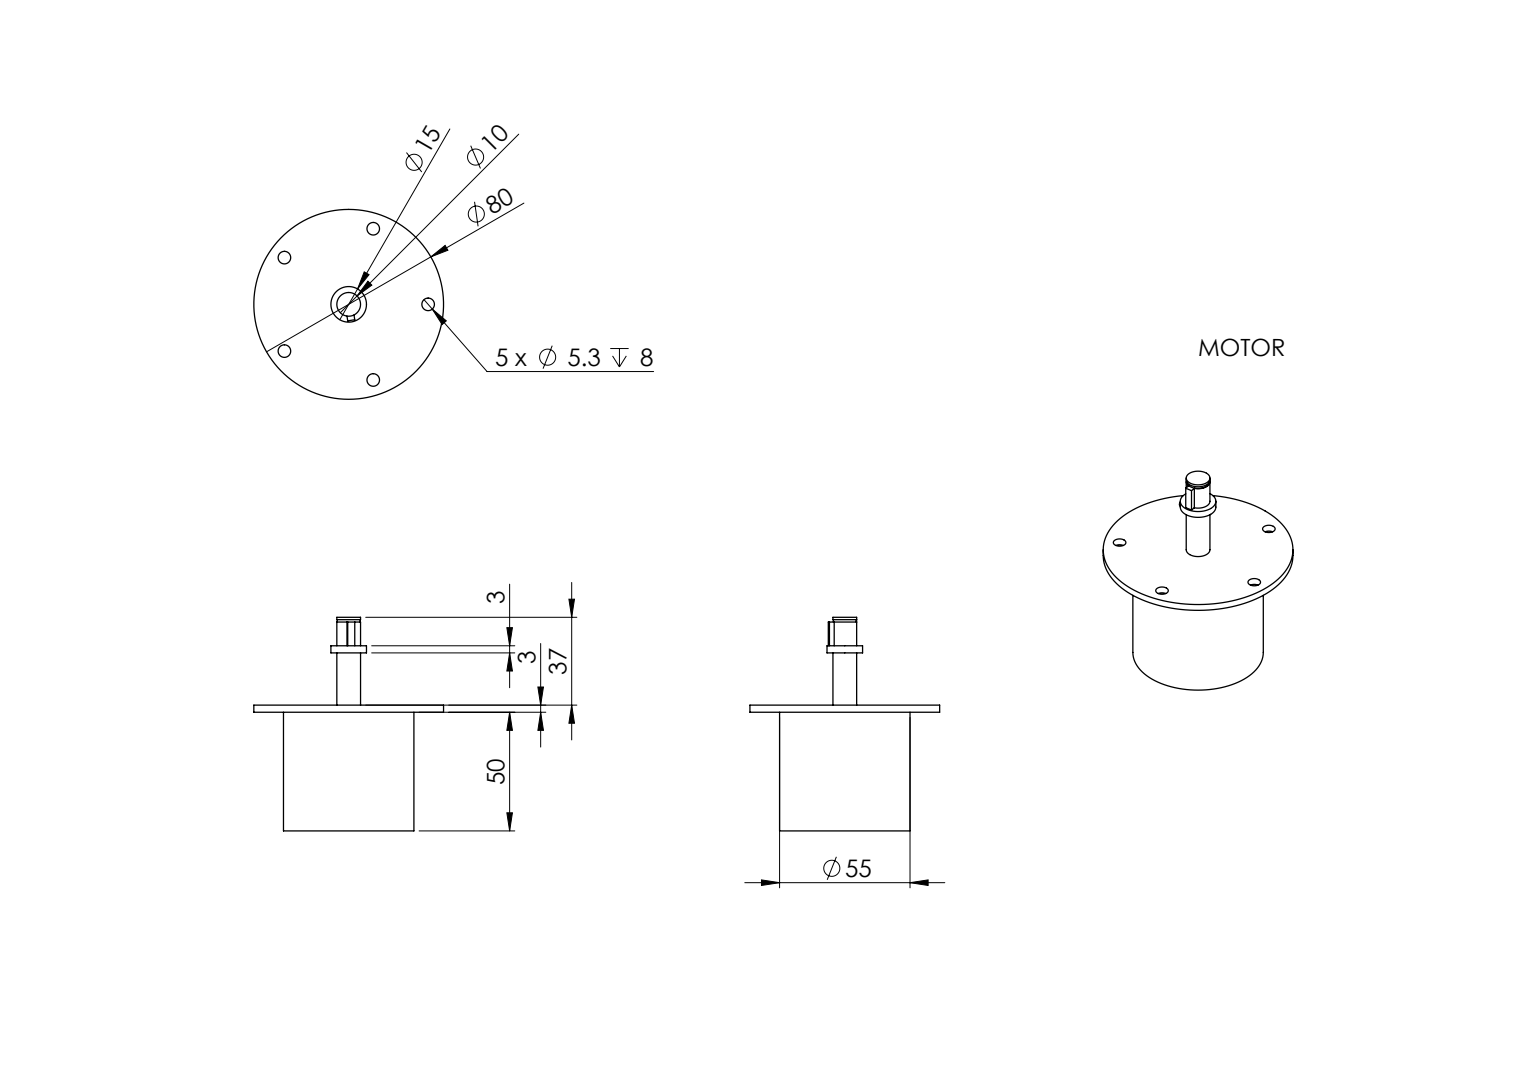
ISO-10303-21;
HEADER;
FILE_DESCRIPTION (('STEP AP214'),
    '1' );
FILE_NAME ('motor.step',
    '2026-10-24T07:08:27',
    ( '' ),
    ( '' ),
    'SwSTEP 2.0',
    'SolidWorks 2026',
    '' );
FILE_SCHEMA (( 'AUTOMOTIVE_DESIGN' ));
ENDSEC;

DATA;
#42=EDGE_CURVE ( 'NONE', #9389, #8733, #2574, .T. ) ;
#55=AXIS2_PLACEMENT_3D ( 'NONE', #9559, #12524, #9279 ) ;
#62=PLANE ( 'NONE',  #8396 ) ;
#84=CARTESIAN_POINT ( 'NONE',  ( -90.00000000009001155, -38.00000000000000000, -1.301042606982603940E-15 ) ) ;
#93=ORIENTED_EDGE ( 'NONE', *, *, #7771, .T. ) ;
#98=FACE_OUTER_BOUND ( 'NONE', #15027, .T. ) ;
#208=DIRECTION ( 'NONE',  ( 0.000000000000000000, 0.000000000000000000, -1.000000000000000000 ) ) ;
#226=CIRCLE ( 'NONE', #3261, 2.649999999999992806 ) ;
#240=CARTESIAN_POINT ( 'NONE',  ( -90.00000000009001155, -38.00000000000000000, -1.301042606982603940E-15 ) ) ;
#245=VECTOR ( 'NONE', #14490, 1000.000000000000000 ) ;
#258=LINE ( 'NONE', #11691, #3125 ) ;
#277=CARTESIAN_POINT ( 'NONE',  ( -90.67999921423555065, 1.000000000000018208, -4.751589320297106234 ) ) ;
#297=AXIS2_PLACEMENT_3D ( 'NONE', #16898, #13842, #16521 ) ;
#342=EDGE_CURVE ( 'NONE', #3837, #6567, #9219, .T. ) ;
#375=EDGE_CURVE ( 'NONE', #12355, #6629, #15146, .T. ) ;
#395=EDGE_CURVE ( 'NONE', #2599, #6420, #1243, .T. ) ;
#405=EDGE_CURVE ( 'NONE', #10887, #2703, #6947, .T. ) ;
#426=ORIENTED_EDGE ( 'NONE', *, *, #405, .T. ) ;
#436=DIRECTION ( 'NONE',  ( 0.000000000000000000, 0.000000000000000000, 1.000000000000000000 ) ) ;
#459=DIRECTION ( 'NONE',  ( 0.000000000000000000, -1.000000000000000000, 0.000000000000000000 ) ) ;
#485=CARTESIAN_POINT ( 'NONE',  ( -90.40159941089927997, 2.081668171172168513E-14, -4.983845695167307355 ) ) ;
#496=EDGE_CURVE ( 'NONE', #11686, #6003, #9891, .T. ) ;
#506=CIRCLE ( 'NONE', #15414, 5.000000000000004441 ) ;
#535=ORIENTED_EDGE ( 'NONE', *, *, #4870, .T. ) ;
#542=VECTOR ( 'NONE', #17182, 1000.000000000000000 ) ;
#547=ORIENTED_EDGE ( 'NONE', *, *, #996, .F. ) ;
#549=LINE ( 'NONE', #1872, #13865 ) ;
#550=ORIENTED_EDGE ( 'NONE', *, *, #5972, .T. ) ;
#563=CARTESIAN_POINT ( 'NONE',  ( -90.00000000009001155, -10.00000000000001599, -1.301042606982603940E-15 ) ) ;
#564=CYLINDRICAL_SURFACE ( 'NONE', #2820, 7.500000000000007105 ) ;
#565=VECTOR ( 'NONE', #11959, 1000.000000000000000 ) ;
#580=EDGE_LOOP ( 'NONE', ( #11778, #1324 ) ) ;
#594=ORIENTED_EDGE ( 'NONE', *, *, #13827, .T. ) ;
#597=CARTESIAN_POINT ( 'NONE',  ( -90.38553543446691663, 1.000000000000018208, -4.784491867360616268 ) ) ;
#598=CARTESIAN_POINT ( 'NONE',  ( -79.64793068852927149, -38.00000000000000000, 34.51039329588763849 ) ) ;
#601=CARTESIAN_POINT ( 'NONE',  ( -90.00000000009001155, -13.00000000000001776, -1.691355389077386325E-15 ) ) ;
#653=ORIENTED_EDGE ( 'NONE', *, *, #10856, .F. ) ;
#671=ORIENTED_EDGE ( 'NONE', *, *, #1460, .F. ) ;
#696=LINE ( 'NONE', #18305, #3229 ) ;
#706=CIRCLE ( 'NONE', #11348, 2.649999999999992806 ) ;
#727=DIRECTION ( 'NONE',  ( 0.000000000000000000, 0.000000000000000000, 1.000000000000000000 ) ) ;
#738=ORIENTED_EDGE ( 'NONE', *, *, #1656, .F. ) ;
#745=STYLED_ITEM ( 'NONE', ( #16686 ), #12609 ) ;
#760=CARTESIAN_POINT ( 'NONE',  ( -94.77031323234206184, 1.000000000000018208, 0.5330212624288541701 ) ) ;
#764=EDGE_CURVE ( 'NONE', #3720, #10887, #3348, .T. ) ;
#776=CARTESIAN_POINT ( 'NONE',  ( -90.00000000009001155, -49.14213562373095812, -5.000000000000005329 ) ) ;
#797=CARTESIAN_POINT ( 'NONE',  ( -90.00000000009001155, -38.00000000000000000, 40.00000000000000000 ) ) ;
#826=UNCERTAINTY_MEASURE_WITH_UNIT (LENGTH_MEASURE( 1.000000000000000082E-05 ), #11317, 'distance_accuracy_value', 'NONE');
#832=CIRCLE ( 'NONE', #6896, 5.000000000000004441 ) ;
#841=AXIS2_PLACEMENT_3D ( 'NONE', #6851, #12669, #4200 ) ;
#846=AXIS2_PLACEMENT_3D ( 'NONE', #6460, #16655, #9411 ) ;
#859=ORIENTED_EDGE ( 'NONE', *, *, #4333, .F. ) ;
#870=AXIS2_PLACEMENT_3D ( 'NONE', #15554, #18308, #10969 ) ;
#874=ORIENTED_EDGE ( 'NONE', *, *, #16459, .T. ) ;
#879=AXIS2_PLACEMENT_3D ( 'NONE', #17078, #7057, #1436 ) ;
#886=CARTESIAN_POINT ( 'NONE',  ( -90.70833251482494575, 2.081668171172168513E-14, -4.949572208642815774 ) ) ;
#892=CIRCLE ( 'NONE', #4521, 2.649999999999992806 ) ;
#913=ORIENTED_EDGE ( 'NONE', *, *, #375, .F. ) ;
#948=ORIENTED_EDGE ( 'NONE', *, *, #9136, .F. ) ;
#949=CARTESIAN_POINT ( 'NONE',  ( -90.00000000009001155, -10.00000000000001599, -1.301042606982603940E-15 ) ) ;
#956=CYLINDRICAL_SURFACE ( 'NONE', #8481, 2.649999999999992806 ) ;
#990=LINE ( 'NONE', #1078, #10722 ) ;
#994=ORIENTED_EDGE ( 'NONE', *, *, #375, .T. ) ;
#996=EDGE_CURVE ( 'NONE', #8916, #9803, #18000, .T. ) ;
#1006=CARTESIAN_POINT ( 'NONE',  ( -117.1020693116506379, -30.00000000000000000, -19.69080595179801207 ) ) ;
#1015=DIRECTION ( 'NONE',  ( 0.000000000000000000, -1.000000000000000000, 0.000000000000000000 ) ) ;
#1020=CARTESIAN_POINT ( 'NONE',  ( -56.50000000009000445, -34.99999999999999289, -2.649999999999610889 ) ) ;
#1075=DIRECTION ( 'NONE',  ( -2.031314180040284764E-16, -1.000000000000000000, -1.301042606982601377E-16 ) ) ;
#1078=CARTESIAN_POINT ( 'NONE',  ( -90.00000000009001155, -49.14213562373095812, -5.000000000000005329 ) ) ;
#1079=DIRECTION ( 'NONE',  ( -0.000000000000000000, 1.000000000000000000, -0.000000000000000000 ) ) ;
#1095=ADVANCED_FACE ( 'NONE', ( #18192 ), #16772, .F. ) ;
#1110=DIRECTION ( 'NONE',  ( 1.000000000000000000, -3.469446951953611231E-16, 0.000000000000000000 ) ) ;
#1121=AXIS2_PLACEMENT_3D ( 'NONE', #7531, #10470, #14766 ) ;
#1127=DIRECTION ( 'NONE',  ( -0.000000000000000000, 1.000000000000000000, 0.000000000000000000 ) ) ;
#1137=DIRECTION ( 'NONE',  ( -1.000000000000000000, 2.312964634635740492E-16, 0.000000000000000000 ) ) ;
#1165=CIRCLE ( 'NONE', #4494, 2.649999999999992806 ) ;
#1174=ORIENTED_EDGE ( 'NONE', *, *, #18088, .F. ) ;
#1182=LINE ( 'NONE', #4037, #9056 ) ;
#1203=CYLINDRICAL_SURFACE ( 'NONE', #14853, 2.649999999999992806 ) ;
#1204=ORIENTED_EDGE ( 'NONE', *, *, #3441, .T. ) ;
#1211=ORIENTED_EDGE ( 'NONE', *, *, #18679, .T. ) ;
#1217=ADVANCED_FACE ( 'NONE', ( #14378 ), #15990, .F. ) ;
#1219=EDGE_CURVE ( 'NONE', #9771, #12239, #15903, .T. ) ;
#1220=CARTESIAN_POINT ( 'NONE',  ( -90.00000000009003998, 1.000000000000018208, -5.746271514173173500E-15 ) ) ;
#1222=CARTESIAN_POINT ( 'NONE',  ( -90.38553543446691663, 1.000000000000018208, -4.784491867360616268 ) ) ;
#1243=LINE ( 'NONE', #7037, #13136 ) ;
#1277=VERTEX_POINT ( 'NONE', #12642 ) ;
#1287=ORIENTED_EDGE ( 'NONE', *, *, #12978, .F. ) ;
#1324=ORIENTED_EDGE ( 'NONE', *, *, #10853, .T. ) ;
#1339=CARTESIAN_POINT ( 'NONE',  ( -90.00000000009003998, 1.000000000000018208, -5.746271514173173500E-15 ) ) ;
#1364=ORIENTED_EDGE ( 'NONE', *, *, #3902, .T. ) ;
#1370=ORIENTED_EDGE ( 'NONE', *, *, #1440, .F. ) ;
#1374=DIRECTION ( 'NONE',  ( 0.000000000000000000, 0.000000000000000000, 1.000000000000000000 ) ) ;
#1382=DIRECTION ( 'NONE',  ( -0.000000000000000000, 1.000000000000000000, -0.000000000000000000 ) ) ;
#1387=DIRECTION ( 'NONE',  ( -2.031314180040284764E-16, -1.000000000000000000, -1.301042606982601377E-16 ) ) ;
#1398=FACE_OUTER_BOUND ( 'NONE', #2904, .T. ) ;
#1402=CYLINDRICAL_SURFACE ( 'NONE', #7880, 7.500000000000007105 ) ;
#1423=CYLINDRICAL_SURFACE ( 'NONE', #16347, 40.00000000000000000 ) ;
#1428=CARTESIAN_POINT ( 'NONE',  ( -90.00000000009001155, -88.00000000000000000, 27.50000000000000000 ) ) ;
#1436=DIRECTION ( 'NONE',  ( 1.000000000000000000, -2.031314180040284764E-16, 0.000000000000000000 ) ) ;
#1440=EDGE_CURVE ( 'NONE', #1277, #9572, #17130, .T. ) ;
#1453=DIRECTION ( 'NONE',  ( -0.000000000000000000, 1.000000000000000000, -0.000000000000000000 ) ) ;
#1456=ORIENTED_EDGE ( 'NONE', *, *, #14822, .T. ) ;
#1460=EDGE_CURVE ( 'NONE', #9528, #7635, #226, .T. ) ;
#1507=VERTEX_POINT ( 'NONE', #9356 ) ;
#1527=CARTESIAN_POINT ( 'NONE',  ( -90.00000000009001155, 2.000000000000001776, -1.301042606982603940E-15 ) ) ;
#1558=FACE_OUTER_BOUND ( 'NONE', #2676, .T. ) ;
#1575=FACE_BOUND ( 'NONE', #4154, .T. ) ;
#1590=CARTESIAN_POINT ( 'NONE',  ( -90.00000000009001155, 2.000000000000001776, -5.000000000000005329 ) ) ;
#1591=DIRECTION ( 'NONE',  ( -0.000000000000000000, 1.000000000000000000, -0.000000000000000000 ) ) ;
#1624=LINE ( 'NONE', #17534, #2968 ) ;
#1645=CARTESIAN_POINT ( 'NONE',  ( -87.43997332177200121, -10.00000000000001954, 6.475821446449875118 ) ) ;
#1656=EDGE_CURVE ( 'NONE', #2709, #2599, #1182, .T. ) ;
#1666=DIRECTION ( 'NONE',  ( 0.1416665029469836024, 0.000000000000000000, 0.9899144417285627995 ) ) ;
#1677=DIRECTION ( 'NONE',  ( -2.031314180040284764E-16, -1.000000000000000000, -1.301042606982601377E-16 ) ) ;
#1681=EDGE_CURVE ( 'NONE', #3221, #14211, #7538, .T. ) ;
#1703=VECTOR ( 'NONE', #11338, 1000.000000000000000 ) ;
#1724=DIRECTION ( 'NONE',  ( 0.000000000000000000, 0.000000000000000000, 1.000000000000000000 ) ) ;
#1737=EDGE_LOOP ( 'NONE', ( #6979, #13598, #3643, #15086 ) ) ;
#1738=FACE_OUTER_BOUND ( 'NONE', #1758, .T. ) ;
#1747=DIRECTION ( 'NONE',  ( 0.1586811557617576196, -1.606889522083438452E-16, 0.9873298794253686506 ) ) ;
#1753=ORIENTED_EDGE ( 'NONE', *, *, #3346, .T. ) ;
#1758=EDGE_LOOP ( 'NONE', ( #16142, #8598, #12894, #6927 ) ) ;
#1761=PRODUCT_DEFINITION_SHAPE ( 'NONE', 'NONE',  #8863 ) ;
#1764=CIRCLE ( 'NONE', #16379, 5.000000000000004441 ) ;
#1770=SHAPE_REPRESENTATION ( 'motor', ( #8017 ), #16855 ) ;
#1775=LINE ( 'NONE', #6150, #565 ) ;
#1791=EDGE_LOOP ( 'NONE', ( #6997, #7591, #14174, #14685 ) ) ;
#1792=EDGE_CURVE ( 'NONE', #10035, #1893, #8740, .T. ) ;
#1793=EDGE_CURVE ( 'NONE', #12173, #10035, #8405, .T. ) ;
#1796=LINE ( 'NONE', #277, #17542 ) ;
#1811=DIRECTION ( 'NONE',  ( 0.000000000000000000, -1.000000000000000000, 0.000000000000000000 ) ) ;
#1816=CYLINDRICAL_SURFACE ( 'NONE', #2469, 2.649999999999992806 ) ;
#1841=DIRECTION ( 'NONE',  ( 0.1416665029469836024, 0.000000000000000000, 0.9899144417285627995 ) ) ;
#1845=EDGE_CURVE ( 'NONE', #1507, #12191, #2986, .T. ) ;
#1867=AXIS2_PLACEMENT_3D ( 'NONE', #14318, #14592, #8682 ) ;
#1872=CARTESIAN_POINT ( 'NONE',  ( -87.43997332177200121, -14.11572627500821042, 6.475821446449874230 ) ) ;
#1875=EDGE_CURVE ( 'NONE', #3186, #11692, #14402, .T. ) ;
#1878=FACE_OUTER_BOUND ( 'NONE', #15547, .T. ) ;
#1893=VERTEX_POINT ( 'NONE', #3072 ) ;
#1906=VECTOR ( 'NONE', #18383, 1000.000000000000000 ) ;
#1909=EDGE_CURVE ( 'NONE', #6825, #12049, #7067, .T. ) ;
#1939=DIRECTION ( 'NONE',  ( 0.000000000000000000, -1.000000000000000000, 0.000000000000000000 ) ) ;
#1958=DIRECTION ( 'NONE',  ( 0.000000000000000000, 0.000000000000000000, 1.000000000000000000 ) ) ;
#1983=PLANE ( 'NONE',  #16615 ) ;
#1991=AXIS2_PLACEMENT_3D ( 'NONE', #7672, #14832, #13501 ) ;
#2033=AXIS2_PLACEMENT_3D ( 'NONE', #1220, #12453, #13874 ) ;
#2039=DIRECTION ( 'NONE',  ( -0.000000000000000000, 1.000000000000000000, -0.000000000000000000 ) ) ;
#2067=ORIENTED_EDGE ( 'NONE', *, *, #7457, .F. ) ;
#2068=AXIS2_PLACEMENT_3D ( 'NONE', #17088, #15644, #2591 ) ;
#2070=DIRECTION ( 'NONE',  ( 0.000000000000000000, 0.000000000000000000, 1.000000000000000000 ) ) ;
#2103=DIRECTION ( 'NONE',  ( -0.000000000000000000, 1.000000000000000000, -0.000000000000000000 ) ) ;
#2124=CARTESIAN_POINT ( 'NONE',  ( -90.67999921423555065, 1.000000000000018208, -4.751589320297106234 ) ) ;
#2132=ORIENTED_EDGE ( 'NONE', *, *, #11827, .T. ) ;
#2149=ORIENTED_EDGE ( 'NONE', *, *, #4870, .F. ) ;
#2151=DIRECTION ( 'NONE',  ( 0.000000000000000000, 0.000000000000000000, -1.000000000000000000 ) ) ;
#2206=APPLICATION_CONTEXT ( 'automotive_design' ) ;
#2210=( LENGTH_UNIT ( ) NAMED_UNIT ( * ) SI_UNIT ( .MILLI., .METRE. ) );
#2233=CYLINDRICAL_SURFACE ( 'NONE', #55, 27.50000000000000000 ) ;
#2243=VERTEX_POINT ( 'NONE', #8204 ) ;
#2258=CARTESIAN_POINT ( 'NONE',  ( -90.00000000009001155, -34.99999999999999289, -1.301042606982603940E-15 ) ) ;
#2285=PLANE ( 'NONE',  #14290 ) ;
#2306=DIRECTION ( 'NONE',  ( 0.000000000000000000, -1.000000000000000000, 0.000000000000000000 ) ) ;
#2360=DIRECTION ( 'NONE',  ( 0.000000000000000000, 0.000000000000000000, -1.000000000000000000 ) ) ;
#2376=ORIENTED_EDGE ( 'NONE', *, *, #9442, .T. ) ;
#2379=ORIENTED_EDGE ( 'NONE', *, *, #1440, .T. ) ;
#2393=DIRECTION ( 'NONE',  ( 0.000000000000000000, 0.000000000000000000, -1.000000000000000000 ) ) ;
#2408=EDGE_CURVE ( 'NONE', #13973, #9267, #18211, .T. ) ;
#2426=ORIENTED_EDGE ( 'NONE', *, *, #14464, .T. ) ;
#2431=CARTESIAN_POINT ( 'NONE',  ( -90.00000000009001155, -38.00000000000000000, -1.301042606982603940E-15 ) ) ;
#2435=CYLINDRICAL_SURFACE ( 'NONE', #8768, 5.000000000000004441 ) ;
#2447=EDGE_CURVE ( 'NONE', #4207, #9803, #7569, .T. ) ;
#2449=CYLINDRICAL_SURFACE ( 'NONE', #2033, 4.799999999999998934 ) ;
#2460=CARTESIAN_POINT ( 'NONE',  ( -85.22968676783801811, 1.821459649775647449E-14, -0.5330212624288650503 ) ) ;
#2469=AXIS2_PLACEMENT_3D ( 'NONE', #16287, #3786, #3247 ) ;
#2533=ORIENTED_EDGE ( 'NONE', *, *, #12490, .F. ) ;
#2574=LINE ( 'NONE', #15729, #1906 ) ;
#2591=DIRECTION ( 'NONE',  ( 0.000000000000000000, 0.000000000000000000, -1.000000000000000000 ) ) ;
#2598=LINE ( 'NONE', #2991, #542 ) ;
#2599=VERTEX_POINT ( 'NONE', #14171 ) ;
#2600=AXIS2_PLACEMENT_3D ( 'NONE', #6445, #3402, #3121 ) ;
#2621=DIRECTION ( 'NONE',  ( 0.000000000000000000, 0.000000000000000000, -1.000000000000000000 ) ) ;
#2640=DIRECTION ( 'NONE',  ( -0.000000000000000000, 1.000000000000000000, -0.000000000000000000 ) ) ;
#2643=AXIS2_PLACEMENT_3D ( 'NONE', #84, #11515, #18741 ) ;
#2674=AXIS2_PLACEMENT_3D ( 'NONE', #15879, #15794, #7202 ) ;
#2676=EDGE_LOOP ( 'NONE', ( #16795, #16322, #14563, #9445, #11509, #13442, #5776, #13951, #6134, #9208, #1287 ) ) ;
#2691=CARTESIAN_POINT ( 'NONE',  ( -90.40196296004810961, -10.00000000000001954, 6.951864913735148477 ) ) ;
#2694=CARTESIAN_POINT ( 'NONE',  ( -90.00000000009001155, -10.00000000000001776, -1.301042606982605912E-15 ) ) ;
#2696=CARTESIAN_POINT ( 'NONE',  ( -90.00000000009001155, -13.00000000000001776, 5.000000000000003553 ) ) ;
#2703=VERTEX_POINT ( 'NONE', #2460 ) ;
#2709=VERTEX_POINT ( 'NONE', #8826 ) ;
#2714=DIRECTION ( 'NONE',  ( 0.000000000000000000, 0.000000000000000000, -1.000000000000000000 ) ) ;
#2719=CARTESIAN_POINT ( 'NONE',  ( -56.50000000009000445, -30.00000000000000000, -2.649999999999610889 ) ) ;
#2730=ADVANCED_FACE ( 'NONE', ( #3029 ), #1402, .T. ) ;
#2747=EDGE_LOOP ( 'NONE', ( #10709, #12559 ) ) ;
#2755=ORIENTED_EDGE ( 'NONE', *, *, #12199, .F. ) ;
#2760=VECTOR ( 'NONE', #6122, 1000.000000000000000 ) ;
#2776=PLANE ( 'NONE',  #879 ) ;
#2808=DIRECTION ( 'NONE',  ( 1.000000000000000000, -2.031314180040284764E-16, 0.000000000000000000 ) ) ;
#2816=DIRECTION ( 'NONE',  ( 0.000000000000000000, -1.000000000000000000, 0.000000000000000000 ) ) ;
#2820=AXIS2_PLACEMENT_3D ( 'NONE', #4849, #11979, #10654 ) ;
#2834=ADVANCED_FACE ( 'NONE', ( #10713 ), #14924, .F. ) ;
#2841=EDGE_CURVE ( 'NONE', #17054, #5933, #17019, .T. ) ;
#2843=VERTEX_POINT ( 'NONE', #1590 ) ;
#2904=EDGE_LOOP ( 'NONE', ( #3062, #8872 ) ) ;
#2923=LINE ( 'NONE', #14544, #7380 ) ;
#2925=ORIENTED_EDGE ( 'NONE', *, *, #496, .F. ) ;
#2932=DIRECTION ( 'NONE',  ( -0.000000000000000000, 1.000000000000000000, -0.000000000000000000 ) ) ;
#2951=DIRECTION ( 'NONE',  ( 0.000000000000000000, 0.000000000000000000, 1.000000000000000000 ) ) ;
#2966=AXIS2_PLACEMENT_3D ( 'NONE', #949, #8074, #6938 ) ;
#2968=VECTOR ( 'NONE', #18162, 1000.000000000000000 ) ;
#2969=VECTOR ( 'NONE', #4414, 1000.000000000000114 ) ;
#2983=CIRCLE ( 'NONE', #13626, 27.50000000000000000 ) ;
#2986=CIRCLE ( 'NONE', #13924, 2.649999999999992806 ) ;
#2991=CARTESIAN_POINT ( 'NONE',  ( -90.38553543446691663, 1.821459649775647449E-14, -4.784491867360616268 ) ) ;
#2992=ORIENTED_EDGE ( 'NONE', *, *, #13827, .F. ) ;
#3011=EDGE_LOOP ( 'NONE', ( #13175, #12108, #8959, #12733 ) ) ;
#3012=VERTEX_POINT ( 'NONE', #18427 ) ;
#3014=CARTESIAN_POINT ( 'NONE',  ( -90.00000000009001155, -34.99999999999999289, -1.301042606982603940E-15 ) ) ;
#3018=CIRCLE ( 'NONE', #17613, 2.649999999999992806 ) ;
#3021=AXIS2_PLACEMENT_3D ( 'NONE', #10352, #13407, #1958 ) ;
#3029=FACE_OUTER_BOUND ( 'NONE', #5506, .T. ) ;
#3038=CARTESIAN_POINT ( 'NONE',  ( -79.64793068852927149, -38.00000000000000000, 31.86039329588764701 ) ) ;
#3042=ORIENTED_EDGE ( 'NONE', *, *, #6050, .T. ) ;
#3053=ORIENTED_EDGE ( 'NONE', *, *, #15279, .F. ) ;
#3057=DIRECTION ( 'NONE',  ( 0.000000000000000000, 0.000000000000000000, -1.000000000000000000 ) ) ;
#3062=ORIENTED_EDGE ( 'NONE', *, *, #5986, .T. ) ;
#3072=CARTESIAN_POINT ( 'NONE',  ( -90.00000000009001155, -34.99999999999999289, -40.00000000000000000 ) ) ;
#3086=FACE_OUTER_BOUND ( 'NONE', #13621, .T. ) ;
#3087=CARTESIAN_POINT ( 'NONE',  ( -56.50000000009000445, -38.00000000000000000, -2.649999999999610889 ) ) ;
#3121=DIRECTION ( 'NONE',  ( 0.000000000000000000, 0.000000000000000000, 1.000000000000000000 ) ) ;
#3125=VECTOR ( 'NONE', #1591, 1000.000000000000000 ) ;
#3137=EDGE_CURVE ( 'NONE', #11692, #6003, #13869, .T. ) ;
#3143=CLOSED_SHELL ( 'NONE', ( #5760, #17055, #1217, #6071, #8539, #14895, #11698, #13435, #3863, #14257, #17180, #2730, #4030, #5733, #6866, #6096, #17687, #8203, #7082, #14045, #6805, #3650, #6257, #5881, #5285, #4348, #10440, #14230, #16768, #10129, #13340, #11631, #4025, #10069, #9467, #2834, #1095 ) ) ;
#3144=DIRECTION ( 'NONE',  ( 0.000000000000000000, -0.000000000000000000, -1.000000000000000000 ) ) ;
#3149=AXIS2_PLACEMENT_3D ( 'NONE', #3748, #9750, #9547 ) ;
#3172=EDGE_CURVE ( 'NONE', #5933, #17054, #16009, .T. ) ;
#3186=VERTEX_POINT ( 'NONE', #6908 ) ;
#3221=VERTEX_POINT ( 'NONE', #9957 ) ;
#3228=CARTESIAN_POINT ( 'NONE',  ( -90.00000000009003998, 1.000000000000018208, -5.746271514173173500E-15 ) ) ;
#3229=VECTOR ( 'NONE', #18217, 999.9999999999998863 ) ;
#3247=DIRECTION ( 'NONE',  ( 0.000000000000000000, 0.000000000000000000, 1.000000000000000000 ) ) ;
#3251=DIRECTION ( 'NONE',  ( -0.000000000000000000, 1.000000000000000000, -0.000000000000000000 ) ) ;
#3261=AXIS2_PLACEMENT_3D ( 'NONE', #15688, #2640, #7023 ) ;
#3270=CARTESIAN_POINT ( 'NONE',  ( -87.43997332177200121, -10.00000000000001954, 6.475821446449876007 ) ) ;
#3276=FACE_OUTER_BOUND ( 'NONE', #6379, .T. ) ;
#3311=CARTESIAN_POINT ( 'NONE',  ( -90.00000000009001155, -13.00000000000001776, -1.301042606982603940E-15 ) ) ;
#3333=VERTEX_POINT ( 'NONE', #6038 ) ;
#3338=DIRECTION ( 'NONE',  ( 0.000000000000000000, 0.000000000000000000, -1.000000000000000000 ) ) ;
#3346=EDGE_CURVE ( 'NONE', #4781, #17733, #5031, .T. ) ;
#3348=CIRCLE ( 'NONE', #297, 4.799999999999998934 ) ;
#3366=PLANE ( 'NONE',  #9913 ) ;
#3382=DIRECTION ( 'NONE',  ( 0.000000000000000000, 0.000000000000000000, -1.000000000000000000 ) ) ;
#3394=DIRECTION ( 'NONE',  ( -0.000000000000000000, 1.000000000000000000, -0.000000000000000000 ) ) ;
#3402=DIRECTION ( 'NONE',  ( -0.000000000000000000, 1.000000000000000000, -0.000000000000000000 ) ) ;
#3410=FACE_OUTER_BOUND ( 'NONE', #13392, .T. ) ;
#3412=EDGE_LOOP ( 'NONE', ( #17004, #11269, #15266, #16917, #10570, #17081, #11839, #550, #6207, #11325, #994, #93 ) ) ;
#3419=CARTESIAN_POINT ( 'NONE',  ( -90.00000000009001155, -49.14213562373095812, -5.000000000000005329 ) ) ;
#3441=EDGE_CURVE ( 'NONE', #9657, #14680, #6769, .T. ) ;
#3442=DIRECTION ( 'NONE',  ( 0.000000000000000000, 0.000000000000000000, -1.000000000000000000 ) ) ;
#3493=EDGE_LOOP ( 'NONE', ( #2149, #2132, #10195, #7456 ) ) ;
#3514=DIRECTION ( 'NONE',  ( 0.9873298794253690946, -1.799126239882931805E-16, -0.1586811557617541224 ) ) ;
#3539=( NAMED_UNIT ( * ) PLANE_ANGLE_UNIT ( ) SI_UNIT ( $, .RADIAN. ) );
#3565=CARTESIAN_POINT ( 'NONE',  ( -79.64793068852898728, -38.00000000000000000, -29.21039329588757383 ) ) ;
#3593=DIRECTION ( 'NONE',  ( 0.000000000000000000, 0.000000000000000000, -1.000000000000000000 ) ) ;
#3614=CYLINDRICAL_SURFACE ( 'NONE', #14823, 4.799999999999998934 ) ;
#3640=SHAPE_REPRESENTATION_RELATIONSHIP ( 'NONE' , 'NONE' ,  #1770, #12609 ) ;
#3643=ORIENTED_EDGE ( 'NONE', *, *, #7218, .F. ) ;
#3649=CARTESIAN_POINT ( 'NONE',  ( -90.00000000009001155, -34.99999999999999289, -5.000000000000005329 ) ) ;
#3650=ADVANCED_FACE ( 'NONE', ( #18078 ), #1983, .T. ) ;
#3653=DIRECTION ( 'NONE',  ( -0.000000000000000000, 1.000000000000000000, -0.000000000000000000 ) ) ;
#3676=CARTESIAN_POINT ( 'NONE',  ( -90.00000000009001155, -38.00000000000000000, 27.50000000000000000 ) ) ;
#3707=CARTESIAN_POINT ( 'NONE',  ( -79.64793068852927149, -34.99999999999999289, 31.86039329588764701 ) ) ;
#3714=CARTESIAN_POINT ( 'NONE',  ( -85.22968676783801811, 1.000000000000018208, -0.5330212624288648282 ) ) ;
#3720=VERTEX_POINT ( 'NONE', #760 ) ;
#3748=CARTESIAN_POINT ( 'NONE',  ( -90.00000000009001155, 2.081668171172168513E-14, -1.301042606982603940E-15 ) ) ;
#3761=CIRCLE ( 'NONE', #3149, 5.000000000000004441 ) ;
#3769=DIRECTION ( 'NONE',  ( 0.000000000000000000, 0.000000000000000000, -1.000000000000000000 ) ) ;
#3786=DIRECTION ( 'NONE',  ( -0.000000000000000000, 1.000000000000000000, -0.000000000000000000 ) ) ;
#3837=VERTEX_POINT ( 'NONE', #7113 ) ;
#3846=VECTOR ( 'NONE', #18525, 1000.000000000000000 ) ;
#3862=FACE_OUTER_BOUND ( 'NONE', #3011, .T. ) ;
#3863=ADVANCED_FACE ( 'NONE', ( #12937 ), #5796, .T. ) ;
#3902=EDGE_CURVE ( 'NONE', #13064, #9389, #5018, .T. ) ;
#3907=CIRCLE ( 'NONE', #6626, 4.799999999999998934 ) ;
#3924=DIRECTION ( 'NONE',  ( 0.000000000000000000, 0.000000000000000000, -1.000000000000000000 ) ) ;
#3925=ORIENTED_EDGE ( 'NONE', *, *, #3441, .F. ) ;
#3927=FACE_OUTER_BOUND ( 'NONE', #1791, .T. ) ;
#3933=ORIENTED_EDGE ( 'NONE', *, *, #7356, .T. ) ;
#3977=ORIENTED_EDGE ( 'NONE', *, *, #42, .T. ) ;
#3987=CARTESIAN_POINT ( 'NONE',  ( -90.00000000009003998, 1.000000000000018208, -5.746271514173173500E-15 ) ) ;
#4025=ADVANCED_FACE ( 'NONE', ( #14928 ), #10538, .F. ) ;
#4029=ORIENTED_EDGE ( 'NONE', *, *, #11169, .T. ) ;
#4030=ADVANCED_FACE ( 'NONE', ( #13314 ), #14731, .T. ) ;
#4034=CARTESIAN_POINT ( 'NONE',  ( -90.00000000009001155, 1.000000000000014655, 5.000000000000003553 ) ) ;
#4037=CARTESIAN_POINT ( 'NONE',  ( -90.40196296004810961, -14.11572627500821042, 6.951864913735147589 ) ) ;
#4046=ORIENTED_EDGE ( 'NONE', *, *, #10927, .F. ) ;
#4047=DIRECTION ( 'NONE',  ( 0.000000000000000000, -1.000000000000000000, 0.000000000000000000 ) ) ;
#4052=EDGE_CURVE ( 'NONE', #9572, #6420, #549, .T. ) ;
#4077=DIRECTION ( 'NONE',  ( 0.000000000000000000, 0.000000000000000000, -1.000000000000000000 ) ) ;
#4081=EDGE_LOOP ( 'NONE', ( #4782, #10644, #2067, #3925 ) ) ;
#4088=( NAMED_UNIT ( * ) SI_UNIT ( $, .STERADIAN. ) SOLID_ANGLE_UNIT ( ) );
#4093=EDGE_CURVE ( 'NONE', #18122, #4173, #10214, .T. ) ;
#4154=EDGE_LOOP ( 'NONE', ( #7724, #2376 ) ) ;
#4162=ORIENTED_EDGE ( 'NONE', *, *, #3137, .T. ) ;
#4173=VERTEX_POINT ( 'NONE', #1020 ) ;
#4174=PLANE ( 'NONE',  #2674 ) ;
#4200=DIRECTION ( 'NONE',  ( 0.000000000000000000, 0.000000000000000000, 1.000000000000000000 ) ) ;
#4205=AXIS2_PLACEMENT_3D ( 'NONE', #7482, #3394, #436 ) ;
#4207=VERTEX_POINT ( 'NONE', #15494 ) ;
#4232=DIRECTION ( 'NONE',  ( 0.000000000000000000, 0.000000000000000000, -1.000000000000000000 ) ) ;
#4271=FACE_BOUND ( 'NONE', #580, .T. ) ;
#4275=AXIS2_PLACEMENT_3D ( 'NONE', #8430, #12612, #2714 ) ;
#4333=EDGE_CURVE ( 'NONE', #4919, #5529, #6864, .T. ) ;
#4348=ADVANCED_FACE ( 'NONE', ( #7291, #1575, #10057, #9865, #12825, #12730, #15954 ), #62, .F. ) ;
#4372=CIRCLE ( 'NONE', #5884, 4.799999999999998934 ) ;
#4394=DIRECTION ( 'NONE',  ( 0.000000000000000000, -1.000000000000000000, 0.000000000000000000 ) ) ;
#4414=DIRECTION ( 'NONE',  ( 0.1586811557617541224, -1.606889522083433522E-16, 0.9873298794253690946 ) ) ;
#4416=CARTESIAN_POINT ( 'NONE',  ( -79.64793068852898728, -30.00000000000000000, -31.86039329588756530 ) ) ;
#4455=EDGE_CURVE ( 'NONE', #5480, #12173, #7489, .T. ) ;
#4469=CARTESIAN_POINT ( 'NONE',  ( -117.1020693116506379, -38.00000000000000000, -17.04080595179801705 ) ) ;
#4494=AXIS2_PLACEMENT_3D ( 'NONE', #10696, #1939, #12223 ) ;
#4511=CARTESIAN_POINT ( 'NONE',  ( -90.00000000009001155, -49.14213562373095812, -1.301042606982603940E-15 ) ) ;
#4521=AXIS2_PLACEMENT_3D ( 'NONE', #8761, #7333, #3057 ) ;
#4540=FACE_OUTER_BOUND ( 'NONE', #4081, .T. ) ;
#4572=AXIS2_PLACEMENT_3D ( 'NONE', #16701, #3653, #9449 ) ;
#4584=CARTESIAN_POINT ( 'NONE',  ( -90.00000000009001155, -38.00000000000000000, 40.00000000000000000 ) ) ;
#4600=DIRECTION ( 'NONE',  ( 0.000000000000000000, -1.000000000000000000, 0.000000000000000000 ) ) ;
#4610=DIRECTION ( 'NONE',  ( -0.000000000000000000, 1.000000000000000000, 0.000000000000000000 ) ) ;
#4653=DIRECTION ( 'NONE',  ( 0.000000000000000000, 0.000000000000000000, -1.000000000000000000 ) ) ;
#4666=VERTEX_POINT ( 'NONE', #9939 ) ;
#4688=EDGE_CURVE ( 'NONE', #3720, #17733, #11276, .T. ) ;
#4696=FACE_OUTER_BOUND ( 'NONE', #12160, .T. ) ;
#4732=LINE ( 'NONE', #15220, #11719 ) ;
#4749=DIRECTION ( 'NONE',  ( 0.000000000000000000, 1.000000000000000000, 0.000000000000000000 ) ) ;
#4781=VERTEX_POINT ( 'NONE', #13806 ) ;
#4782=ORIENTED_EDGE ( 'NONE', *, *, #8424, .F. ) ;
#4783=VECTOR ( 'NONE', #8234, 1000.000000000000000 ) ;
#4794=DIRECTION ( 'NONE',  ( 0.9873298794253685395, 0.000000000000000000, -0.1586811557617575918 ) ) ;
#4829=CARTESIAN_POINT ( 'NONE',  ( -56.50000000009000445, -34.99999999999999289, 2.650000000000374278 ) ) ;
#4830=ORIENTED_EDGE ( 'NONE', *, *, #14658, .F. ) ;
#4849=CARTESIAN_POINT ( 'NONE',  ( -90.00000000009001155, -13.00000000000001776, -1.691355389077386325E-15 ) ) ;
#4866=LINE ( 'NONE', #776, #6562 ) ;
#4870=EDGE_CURVE ( 'NONE', #13797, #9771, #832, .T. ) ;
#4876=ORIENTED_EDGE ( 'NONE', *, *, #18327, .F. ) ;
#4919=VERTEX_POINT ( 'NONE', #13139 ) ;
#4934=DIRECTION ( 'NONE',  ( 0.000000000000000000, -1.000000000000000000, 0.000000000000000000 ) ) ;
#4956=DIRECTION ( 'NONE',  ( -0.9873298794253690946, 1.799126239882931805E-16, 0.1586811557617541224 ) ) ;
#4972=CARTESIAN_POINT ( 'NONE',  ( -90.00000000009001155, 2.000000000000001776, 5.000000000000003553 ) ) ;
#4973=ORIENTED_EDGE ( 'NONE', *, *, #1460, .T. ) ;
#4978=CARTESIAN_POINT ( 'NONE',  ( -90.67999921423555065, 1.821459649775647449E-14, -4.751589320297106234 ) ) ;
#4993=EDGE_CURVE ( 'NONE', #3333, #4781, #1796, .T. ) ;
#5018=CIRCLE ( 'NONE', #11473, 27.50000000000000000 ) ;
#5031=CIRCLE ( 'NONE', #7781, 4.799999999999998934 ) ;
#5046=FILL_AREA_STYLE_COLOUR ( '', #8635 ) ;
#5054=ORIENTED_EDGE ( 'NONE', *, *, #4688, .F. ) ;
#5061=CARTESIAN_POINT ( 'NONE',  ( -79.64793068852927149, -38.00000000000000000, 29.21039329588765554 ) ) ;
#5141=CARTESIAN_POINT ( 'NONE',  ( -79.64793068852927149, -30.00000000000000000, 31.86039329588764701 ) ) ;
#5161=VECTOR ( 'NONE', #1382, 1000.000000000000000 ) ;
#5192=CARTESIAN_POINT ( 'NONE',  ( -90.00000000009001155, -38.00000000000000000, -1.301042606982603940E-15 ) ) ;
#5197=DIRECTION ( 'NONE',  ( 0.1586811557617541502, -1.606889522083424400E-16, 0.9873298794253692057 ) ) ;
#5212=DIRECTION ( 'NONE',  ( 0.9938152567191714803, 0.000000000000000000, -0.1110460963393456596 ) ) ;
#5215=ORIENTED_EDGE ( 'NONE', *, *, #15890, .F. ) ;
#5240=DIRECTION ( 'NONE',  ( 0.000000000000000000, -1.000000000000000000, 0.000000000000000000 ) ) ;
#5267=AXIS2_PLACEMENT_3D ( 'NONE', #7797, #1811, #9317 ) ;
#5285=ADVANCED_FACE ( 'NONE', ( #5805 ), #1423, .T. ) ;
#5301=EDGE_LOOP ( 'NONE', ( #18311, #7953 ) ) ;
#5326=PRODUCT_DEFINITION_FORMATION_WITH_SPECIFIED_SOURCE ( 'ANY', '', #17887, .NOT_KNOWN. ) ;
#5381=UNCERTAINTY_MEASURE_WITH_UNIT (LENGTH_MEASURE( 1.000000000000000082E-05 ), #13730, 'distance_accuracy_value', 'NONE');
#5382=FACE_OUTER_BOUND ( 'NONE', #3412, .T. ) ;
#5414=CARTESIAN_POINT ( 'NONE',  ( -90.00000000009001155, -38.00000000000000000, -40.00000000000000000 ) ) ;
#5445=STYLED_ITEM('',(#18890),#15813);
#5468=CARTESIAN_POINT ( 'NONE',  ( -117.1020693116508085, -38.00000000000000000, 19.69080595179778115 ) ) ;
#5480=VERTEX_POINT ( 'NONE', #5414 ) ;
#5506=EDGE_LOOP ( 'NONE', ( #859, #1211, #18336, #17947 ) ) ;
#5529=VERTEX_POINT ( 'NONE', #15227 ) ;
#5580=CARTESIAN_POINT ( 'NONE',  ( -56.50000000009000445, -30.00000000000000000, 2.650000000000374278 ) ) ;
#5588=EDGE_CURVE ( 'NONE', #3333, #3720, #3907, .T. ) ;
#5647=ORIENTED_EDGE ( 'NONE', *, *, #7749, .T. ) ;
#5662=VECTOR ( 'NONE', #2039, 1000.000000000000000 ) ;
#5687=DIRECTION ( 'NONE',  ( -0.9967691390334607604, -0.000000000000000000, 0.08031988216184954288 ) ) ;
#5731=EDGE_LOOP ( 'NONE', ( #12461, #6385, #874, #10336 ) ) ;
#5732=CIRCLE ( 'NONE', #12415, 40.00000000000000000 ) ;
#5733=ADVANCED_FACE ( 'NONE', ( #10158, #4271, #10071, #17218, #1398, #15964, #8631 ), #4174, .T. ) ;
#5760=ADVANCED_FACE ( 'NONE', ( #4540 ), #16444, .F. ) ;
#5776=ORIENTED_EDGE ( 'NONE', *, *, #10124, .F. ) ;
#5796=CYLINDRICAL_SURFACE ( 'NONE', #2643, 40.00000000000000000 ) ;
#5805=FACE_OUTER_BOUND ( 'NONE', #8442, .T. ) ;
#5858=EDGE_CURVE ( 'NONE', #1277, #10958, #1775, .T. ) ;
#5866=AXIS2_PLACEMENT_3D ( 'NONE', #2124, #7928, #1841 ) ;
#5881=ADVANCED_FACE ( 'NONE', ( #5382 ), #2435, .T. ) ;
#5884=AXIS2_PLACEMENT_3D ( 'NONE', #17471, #8805, #8893 ) ;
#5896=DIRECTION ( 'NONE',  ( 0.9938152567191714803, 0.000000000000000000, -0.1110460963393456596 ) ) ;
#5924=AXIS2_PLACEMENT_3D ( 'NONE', #13505, #17882, #10642 ) ;
#5933=VERTEX_POINT ( 'NONE', #14052 ) ;
#5972=EDGE_CURVE ( 'NONE', #12239, #2843, #1764, .T. ) ;
#5986=EDGE_CURVE ( 'NONE', #12173, #5480, #5732, .T. ) ;
#6003=VERTEX_POINT ( 'NONE', #15487 ) ;
#6008=FACE_OUTER_BOUND ( 'NONE', #3493, .T. ) ;
#6032=AXIS2_PLACEMENT_3D ( 'NONE', #15858, #13102, #2808 ) ;
#6038=CARTESIAN_POINT ( 'NONE',  ( -90.67999921423555065, 1.000000000000018208, -4.751589320297106234 ) ) ;
#6048=ORIENTED_EDGE ( 'NONE', *, *, #17158, .F. ) ;
#6050=EDGE_CURVE ( 'NONE', #9528, #4173, #7004, .T. ) ;
#6052=CARTESIAN_POINT ( 'NONE',  ( -90.67999921423555065, 1.000000000000018208, -4.751589320297106234 ) ) ;
#6071=ADVANCED_FACE ( 'NONE', ( #17195 ), #1203, .F. ) ;
#6073=DIRECTION ( 'NONE',  ( 0.9938152567191715914, 0.000000000000000000, -0.1110460963393456735 ) ) ;
#6090=ORIENTED_EDGE ( 'NONE', *, *, #11169, .F. ) ;
#6096=ADVANCED_FACE ( 'NONE', ( #17108, #10048 ), #9954, .F. ) ;
#6122=DIRECTION ( 'NONE',  ( -0.000000000000000000, 1.000000000000000000, -0.000000000000000000 ) ) ;
#6134=ORIENTED_EDGE ( 'NONE', *, *, #3346, .F. ) ;
#6150=CARTESIAN_POINT ( 'NONE',  ( -87.76214430591549842, -14.11572627500821042, 4.471241649927994111 ) ) ;
#6199=EDGE_LOOP ( 'NONE', ( #17961, #17758, #9700, #6048 ) ) ;
#6207=ORIENTED_EDGE ( 'NONE', *, *, #11827, .F. ) ;
#6224=ORIENTED_EDGE ( 'NONE', *, *, #17736, .F. ) ;
#6257=ADVANCED_FACE ( 'NONE', ( #4696 ), #14901, .T. ) ;
#6308=DIRECTION ( 'NONE',  ( 0.000000000000000000, -0.000000000000000000, -1.000000000000000000 ) ) ;
#6363=PLANE ( 'NONE',  #16880 ) ;
#6373=CIRCLE ( 'NONE', #17032, 5.000000000000004441 ) ;
#6374=CARTESIAN_POINT ( 'NONE',  ( -117.1020693116508085, -34.99999999999999289, 19.69080595179778115 ) ) ;
#6379=EDGE_LOOP ( 'NONE', ( #7991, #10078, #2992, #10698 ) ) ;
#6385=ORIENTED_EDGE ( 'NONE', *, *, #17962, .T. ) ;
#6392=ORIENTED_EDGE ( 'NONE', *, *, #7018, .F. ) ;
#6420=VERTEX_POINT ( 'NONE', #18312 ) ;
#6445=CARTESIAN_POINT ( 'NONE',  ( -56.50000000009000445, -30.00000000000000000, 3.817814120399276590E-13 ) ) ;
#6460=CARTESIAN_POINT ( 'NONE',  ( -117.1020693116508085, -38.00000000000000000, 19.69080595179778115 ) ) ;
#6507=LINE ( 'NONE', #15560, #16846 ) ;
#6548=CARTESIAN_POINT ( 'NONE',  ( -117.1020693116506379, -34.99999999999999289, -22.34080595179800355 ) ) ;
#6562=VECTOR ( 'NONE', #16489, 1000.000000000000000 ) ;
#6567=VERTEX_POINT ( 'NONE', #13538 ) ;
#6626=AXIS2_PLACEMENT_3D ( 'NONE', #3987, #11218, #5212 ) ;
#6629=VERTEX_POINT ( 'NONE', #485 ) ;
#6655=ORIENTED_EDGE ( 'NONE', *, *, #12272, .F. ) ;
#6659=ORIENTED_EDGE ( 'NONE', *, *, #6050, .F. ) ;
#6665=DIRECTION ( 'NONE',  ( 0.000000000000000000, 0.000000000000000000, 1.000000000000000000 ) ) ;
#6689=EDGE_CURVE ( 'NONE', #14440, #10477, #16706, .T. ) ;
#6698=DIRECTION ( 'NONE',  ( -2.031314180040284764E-16, -1.000000000000000000, -1.301042606982601377E-16 ) ) ;
#6723=AXIS2_PLACEMENT_3D ( 'NONE', #10571, #1127, #11213 ) ;
#6736=CARTESIAN_POINT ( 'NONE',  ( -90.00000000009001155, -34.99999999999999289, 40.00000000000000000 ) ) ;
#6751=EDGE_CURVE ( 'NONE', #9771, #12049, #13365, .T. ) ;
#6769=LINE ( 'NONE', #15088, #5662 ) ;
#6805=ADVANCED_FACE ( 'NONE', ( #18006 ), #2285, .T. ) ;
#6809=CARTESIAN_POINT ( 'NONE',  ( -90.00000000009001155, -49.14213562373095812, -1.301042606982603940E-15 ) ) ;
#6820=CARTESIAN_POINT ( 'NONE',  ( -90.00000000009001155, 2.000000000000001776, -1.301042606982603940E-15 ) ) ;
#6825=VERTEX_POINT ( 'NONE', #886 ) ;
#6837=ORIENTED_EDGE ( 'NONE', *, *, #18205, .T. ) ;
#6851=CARTESIAN_POINT ( 'NONE',  ( -117.1020693116506379, -30.00000000000000000, -19.69080595179801207 ) ) ;
#6859=CIRCLE ( 'NONE', #13241, 2.649999999999992806 ) ;
#6864=CIRCLE ( 'NONE', #10813, 7.500000000000007105 ) ;
#6866=ADVANCED_FACE ( 'NONE', ( #3927 ), #7135, .T. ) ;
#6876=DIRECTION ( 'NONE',  ( 2.031314180040284764E-16, 1.000000000000000000, 1.301042606982601623E-16 ) ) ;
#6896=AXIS2_PLACEMENT_3D ( 'NONE', #8652, #14459, #14560 ) ;
#6908=CARTESIAN_POINT ( 'NONE',  ( -117.1020693116506379, -38.00000000000000000, -22.34080595179800355 ) ) ;
#6927=ORIENTED_EDGE ( 'NONE', *, *, #5858, .F. ) ;
#6938=DIRECTION ( 'NONE',  ( 1.000000000000000000, -3.469446951953611231E-16, 0.000000000000000000 ) ) ;
#6947=LINE ( 'NONE', #3714, #13447 ) ;
#6979=ORIENTED_EDGE ( 'NONE', *, *, #14464, .F. ) ;
#6985=DIRECTION ( 'NONE',  ( 0.000000000000000000, 0.000000000000000000, -1.000000000000000000 ) ) ;
#6997=ORIENTED_EDGE ( 'NONE', *, *, #12752, .F. ) ;
#7004=LINE ( 'NONE', #2719, #18496 ) ;
#7018=EDGE_CURVE ( 'NONE', #10477, #14440, #16415, .T. ) ;
#7019=FACE_OUTER_BOUND ( 'NONE', #12880, .T. ) ;
#7023=DIRECTION ( 'NONE',  ( 0.000000000000000000, 0.000000000000000000, -1.000000000000000000 ) ) ;
#7028=ORIENTED_EDGE ( 'NONE', *, *, #7697, .T. ) ;
#7037=CARTESIAN_POINT ( 'NONE',  ( -90.40196296004810961, 1.745901168134654787E-14, 6.951864913735149365 ) ) ;
#7050=DIRECTION ( 'NONE',  ( -0.000000000000000000, 1.000000000000000000, -0.000000000000000000 ) ) ;
#7051=EDGE_LOOP ( 'NONE', ( #1370, #7896, #653, #17908 ) ) ;
#7057=DIRECTION ( 'NONE',  ( -2.031314180040284764E-16, -1.000000000000000000, -1.301042606982601377E-16 ) ) ;
#7063=DIRECTION ( 'NONE',  ( -0.9873298794253686506, 1.799126239882929340E-16, 0.1586811557617576196 ) ) ;
#7067=LINE ( 'NONE', #12891, #245 ) ;
#7082=ADVANCED_FACE ( 'NONE', ( #11625 ), #8754, .F. ) ;
#7096=DIRECTION ( 'NONE',  ( 1.000000000000000000, -2.312964634635740492E-16, 0.000000000000000000 ) ) ;
#7113=CARTESIAN_POINT ( 'NONE',  ( -79.64793068852898728, -34.99999999999999289, -29.21039329588757383 ) ) ;
#7129=DIRECTION ( 'NONE',  ( 0.000000000000000000, -1.000000000000000000, 0.000000000000000000 ) ) ;
#7135=CYLINDRICAL_SURFACE ( 'NONE', #11252, 5.000000000000004441 ) ;
#7151=CARTESIAN_POINT ( 'NONE',  ( -90.72413394419160682, -10.00000000000001954, 4.947285117213268357 ) ) ;
#7172=AXIS2_PLACEMENT_3D ( 'NONE', #15021, #15118, #2070 ) ;
#7202=DIRECTION ( 'NONE',  ( 0.000000000000000000, -0.000000000000000000, -1.000000000000000000 ) ) ;
#7205=ORIENTED_EDGE ( 'NONE', *, *, #17403, .T. ) ;
#7206=CIRCLE ( 'NONE', #2966, 5.000000000000004441 ) ;
#7218=EDGE_CURVE ( 'NONE', #9150, #2599, #12442, .T. ) ;
#7224=ORIENTED_EDGE ( 'NONE', *, *, #7457, .T. ) ;
#7235=ORIENTED_EDGE ( 'NONE', *, *, #8831, .T. ) ;
#7251=ORIENTED_EDGE ( 'NONE', *, *, #11860, .F. ) ;
#7252=AXIS2_PLACEMENT_3D ( 'NONE', #563, #16183, #17702 ) ;
#7258=DIRECTION ( 'NONE',  ( -0.000000000000000000, 1.000000000000000000, -0.000000000000000000 ) ) ;
#7283=DIRECTION ( 'NONE',  ( -0.000000000000000000, 1.000000000000000000, -0.000000000000000000 ) ) ;
#7291=FACE_BOUND ( 'NONE', #15923, .T. ) ;
#7309=DIRECTION ( 'NONE',  ( 2.031314180040284764E-16, 1.000000000000000000, 1.301042606982601377E-16 ) ) ;
#7333=DIRECTION ( 'NONE',  ( -0.000000000000000000, 1.000000000000000000, -0.000000000000000000 ) ) ;
#7356=EDGE_CURVE ( 'NONE', #7635, #18122, #10143, .T. ) ;
#7380=VECTOR ( 'NONE', #7309, 1000.000000000000000 ) ;
#7456=ORIENTED_EDGE ( 'NONE', *, *, #1219, .F. ) ;
#7457=EDGE_CURVE ( 'NONE', #14680, #2243, #1165, .T. ) ;
#7482=CARTESIAN_POINT ( 'NONE',  ( -79.64793068852927149, -30.00000000000000000, 31.86039329588764701 ) ) ;
#7489=CIRCLE ( 'NONE', #14477, 40.00000000000000000 ) ;
#7505=DIRECTION ( 'NONE',  ( 0.000000000000000000, -1.000000000000000000, 0.000000000000000000 ) ) ;
#7531=CARTESIAN_POINT ( 'NONE',  ( -56.50000000009000445, -34.99999999999999289, 3.817814120399276590E-13 ) ) ;
#7532=CIRCLE ( 'NONE', #18183, 5.000000000000004441 ) ;
#7538=CIRCLE ( 'NONE', #870, 7.500000000000007105 ) ;
#7569=CIRCLE ( 'NONE', #12437, 2.649999999999992806 ) ;
#7589=DIRECTION ( 'NONE',  ( 2.031314180040284764E-16, 1.000000000000000000, 1.301042606982601623E-16 ) ) ;
#7591=ORIENTED_EDGE ( 'NONE', *, *, #6689, .T. ) ;
#7635=VERTEX_POINT ( 'NONE', #9652 ) ;
#7672=CARTESIAN_POINT ( 'NONE',  ( -56.50000000009000445, -34.99999999999999289, 3.817814120399276590E-13 ) ) ;
#7679=CYLINDRICAL_SURFACE ( 'NONE', #5924, 27.50000000000000000 ) ;
#7697=EDGE_CURVE ( 'NONE', #3012, #4207, #9459, .T. ) ;
#7711=LINE ( 'NONE', #14877, #8576 ) ;
#7724=ORIENTED_EDGE ( 'NONE', *, *, #2447, .T. ) ;
#7726=MECHANICAL_DESIGN_GEOMETRIC_PRESENTATION_REPRESENTATION('',(#745),#11701);
#7749=EDGE_CURVE ( 'NONE', #4666, #6629, #2598, .T. ) ;
#7771=EDGE_CURVE ( 'NONE', #6629, #13789, #7532, .T. ) ;
#7781=AXIS2_PLACEMENT_3D ( 'NONE', #17664, #4610, #10418 ) ;
#7788=AXIS2_PLACEMENT_3D ( 'NONE', #4511, #10407, #10491 ) ;
#7791=AXIS2_PLACEMENT_3D ( 'NONE', #18711, #8437, #1110 ) ;
#7797=CARTESIAN_POINT ( 'NONE',  ( -79.64793068852898728, -34.99999999999999289, -31.86039329588756530 ) ) ;
#7880=AXIS2_PLACEMENT_3D ( 'NONE', #11690, #17494, #1137 ) ;
#7896=ORIENTED_EDGE ( 'NONE', *, *, #5858, .T. ) ;
#7913=CIRCLE ( 'NONE', #4572, 2.649999999999992806 ) ;
#7928=DIRECTION ( 'NONE',  ( 0.9899144417285629105, 0.000000000000000000, -0.1416665029469836301 ) ) ;
#7953=ORIENTED_EDGE ( 'NONE', *, *, #11072, .F. ) ;
#7976=DIRECTION ( 'NONE',  ( 0.000000000000000000, 0.000000000000000000, -1.000000000000000000 ) ) ;
#7979=FACE_OUTER_BOUND ( 'NONE', #14626, .T. ) ;
#7988=CIRCLE ( 'NONE', #17125, 2.649999999999992806 ) ;
#7991=ORIENTED_EDGE ( 'NONE', *, *, #18603, .T. ) ;
#8017=AXIS2_PLACEMENT_3D ( 'NONE', #12801, #14324, #9934 ) ;
#8057=CARTESIAN_POINT ( 'NONE',  ( -117.1020693116508085, -38.00000000000000000, 17.04080595179778967 ) ) ;
#8074=DIRECTION ( 'NONE',  ( -2.031314180040284764E-16, -1.000000000000000000, -1.301042606982601377E-16 ) ) ;
#8085=DIRECTION ( 'NONE',  ( -0.000000000000000000, 1.000000000000000000, -0.000000000000000000 ) ) ;
#8087=VECTOR ( 'NONE', #13450, 1000.000000000000000 ) ;
#8094=ORIENTED_EDGE ( 'NONE', *, *, #3172, .T. ) ;
#8099=DIRECTION ( 'NONE',  ( 0.000000000000000000, 0.000000000000000000, 1.000000000000000000 ) ) ;
#8203=ADVANCED_FACE ( 'NONE', ( #12678, #12965 ), #2776, .T. ) ;
#8204=CARTESIAN_POINT ( 'NONE',  ( -79.64793068852927149, -34.99999999999999289, 29.21039329588765554 ) ) ;
#8234=DIRECTION ( 'NONE',  ( -0.000000000000000000, 1.000000000000000000, -0.000000000000000000 ) ) ;
#8245=DIRECTION ( 'NONE',  ( 0.000000000000000000, 0.000000000000000000, -1.000000000000000000 ) ) ;
#8248=DIRECTION ( 'NONE',  ( -0.000000000000000000, 1.000000000000000000, -0.000000000000000000 ) ) ;
#8355=EDGE_LOOP ( 'NONE', ( #16837, #3053 ) ) ;
#8396=AXIS2_PLACEMENT_3D ( 'NONE', #3014, #2816, #8622 ) ;
#8405=LINE ( 'NONE', #4584, #13627 ) ;
#8412=CIRCLE ( 'NONE', #11752, 7.500000000000007105 ) ;
#8424=EDGE_CURVE ( 'NONE', #9696, #9657, #892, .T. ) ;
#8430=CARTESIAN_POINT ( 'NONE',  ( -117.1020693116508085, -34.99999999999999289, 19.69080595179778115 ) ) ;
#8431=VECTOR ( 'NONE', #2103, 1000.000000000000000 ) ;
#8437=DIRECTION ( 'NONE',  ( -2.031314180040284764E-16, -1.000000000000000000, -1.301042606982601377E-16 ) ) ;
#8442=EDGE_LOOP ( 'NONE', ( #10159, #17865, #10011, #9570 ) ) ;
#8481=AXIS2_PLACEMENT_3D ( 'NONE', #12560, #13800, #6665 ) ;
#8539=ADVANCED_FACE ( 'NONE', ( #12366 ), #956, .F. ) ;
#8544=EDGE_LOOP ( 'NONE', ( #17685, #4046, #13661, #17051 ) ) ;
#8576=VECTOR ( 'NONE', #11995, 1000.000000000000000 ) ;
#8598=ORIENTED_EDGE ( 'NONE', *, *, #16836, .T. ) ;
#8600=SHAPE_DEFINITION_REPRESENTATION ( #1761, #1770 ) ;
#8622=DIRECTION ( 'NONE',  ( 0.000000000000000000, -0.000000000000000000, -1.000000000000000000 ) ) ;
#8627=ORIENTED_EDGE ( 'NONE', *, *, #17736, .T. ) ;
#8631=FACE_BOUND ( 'NONE', #2747, .T. ) ;
#8635=COLOUR_RGB ( '',0.8941176470588234615, 0.8941176470588234615, 0.8941176470588234615 ) ;
#8652=CARTESIAN_POINT ( 'NONE',  ( -90.00000000009001155, 1.000000000000014655, -1.301042606982603940E-15 ) ) ;
#8682=DIRECTION ( 'NONE',  ( 0.000000000000000000, 0.000000000000000000, 1.000000000000000000 ) ) ;
#8733=VERTEX_POINT ( 'NONE', #13039 ) ;
#8740=CIRCLE ( 'NONE', #2068, 40.00000000000000000 ) ;
#8743=ORIENTED_EDGE ( 'NONE', *, *, #4052, .T. ) ;
#8754=PLANE ( 'NONE',  #9729 ) ;
#8761=CARTESIAN_POINT ( 'NONE',  ( -79.64793068852927149, -38.00000000000000000, 31.86039329588764701 ) ) ;
#8768=AXIS2_PLACEMENT_3D ( 'NONE', #6809, #8248, #727 ) ;
#8781=LINE ( 'NONE', #13359, #8087 ) ;
#8805=DIRECTION ( 'NONE',  ( -0.000000000000000000, 1.000000000000000000, 0.000000000000000000 ) ) ;
#8807=ORIENTED_EDGE ( 'NONE', *, *, #7356, .F. ) ;
#8824=VECTOR ( 'NONE', #7063, 999.9999999999998863 ) ;
#8826=CARTESIAN_POINT ( 'NONE',  ( -90.40196296004810961, -10.00000000000001954, 6.951864913735149365 ) ) ;
#8831=EDGE_CURVE ( 'NONE', #9657, #9696, #3018, .T. ) ;
#8863=PRODUCT_DEFINITION ( 'UNKNOWN', '', #5326, #12838 ) ;
#8872=ORIENTED_EDGE ( 'NONE', *, *, #4455, .T. ) ;
#8893=DIRECTION ( 'NONE',  ( 0.9938152567191714803, 0.000000000000000000, -0.1110460963393456596 ) ) ;
#8916=VERTEX_POINT ( 'NONE', #8057 ) ;
#8954=DIRECTION ( 'NONE',  ( 0.000000000000000000, 1.000000000000000000, 0.000000000000000000 ) ) ;
#8959=ORIENTED_EDGE ( 'NONE', *, *, #14658, .T. ) ;
#8993=AXIS2_PLACEMENT_3D ( 'NONE', #13095, #14416, #9946 ) ;
#9056=VECTOR ( 'NONE', #6876, 1000.000000000000000 ) ;
#9111=ORIENTED_EDGE ( 'NONE', *, *, #18205, .F. ) ;
#9132=CARTESIAN_POINT ( 'NONE',  ( -94.77031323234206184, 1.821459649775647449E-14, 0.5330212624288541701 ) ) ;
#9136=EDGE_CURVE ( 'NONE', #2843, #12239, #6373, .T. ) ;
#9150=VERTEX_POINT ( 'NONE', #9775 ) ;
#9155=ORIENTED_EDGE ( 'NONE', *, *, #4093, .T. ) ;
#9196=ORIENTED_EDGE ( 'NONE', *, *, #1845, .T. ) ;
#9205=DIRECTION ( 'NONE',  ( 0.000000000000000000, -1.000000000000000000, 0.000000000000000000 ) ) ;
#9208=ORIENTED_EDGE ( 'NONE', *, *, #18603, .F. ) ;
#9213=DIRECTION ( 'NONE',  ( -0.000000000000000000, 1.000000000000000000, -0.000000000000000000 ) ) ;
#9219=CIRCLE ( 'NONE', #5267, 2.649999999999992806 ) ;
#9251=EDGE_LOOP ( 'NONE', ( #17349, #9196 ) ) ;
#9267=VERTEX_POINT ( 'NONE', #17954 ) ;
#9279=DIRECTION ( 'NONE',  ( 0.000000000000000000, 0.000000000000000000, 1.000000000000000000 ) ) ;
#9284=CIRCLE ( 'NONE', #16900, 2.649999999999992806 ) ;
#9317=DIRECTION ( 'NONE',  ( 0.000000000000000000, 0.000000000000000000, -1.000000000000000000 ) ) ;
#9333=DIRECTION ( 'NONE',  ( 0.1586811557617541224, 0.000000000000000000, 0.9873298794253690946 ) ) ;
#9346=ORIENTED_EDGE ( 'NONE', *, *, #12828, .F. ) ;
#9356=CARTESIAN_POINT ( 'NONE',  ( -79.64793068852898728, -38.00000000000000000, -34.51039329588756033 ) ) ;
#9388=CARTESIAN_POINT ( 'NONE',  ( -90.00000000009001155, 2.000000000000001776, -1.301042606982603940E-15 ) ) ;
#9389=VERTEX_POINT ( 'NONE', #17296 ) ;
#9411=DIRECTION ( 'NONE',  ( 0.000000000000000000, 0.000000000000000000, -1.000000000000000000 ) ) ;
#9416=ORIENTED_EDGE ( 'NONE', *, *, #10927, .T. ) ;
#9429=CARTESIAN_POINT ( 'NONE',  ( -90.00000000009001155, 1.000000000000014655, -1.301042606982603940E-15 ) ) ;
#9442=EDGE_CURVE ( 'NONE', #9803, #4207, #14000, .T. ) ;
#9445=ORIENTED_EDGE ( 'NONE', *, *, #18667, .F. ) ;
#9449=DIRECTION ( 'NONE',  ( 0.000000000000000000, 0.000000000000000000, -1.000000000000000000 ) ) ;
#9459=LINE ( 'NONE', #18402, #4783 ) ;
#9467=ADVANCED_FACE ( 'NONE', ( #11078 ), #12715, .F. ) ;
#9494=LINE ( 'NONE', #18546, #11163 ) ;
#9521=DIRECTION ( 'NONE',  ( -0.000000000000000000, 1.000000000000000000, -0.000000000000000000 ) ) ;
#9528=VERTEX_POINT ( 'NONE', #3087 ) ;
#9547=DIRECTION ( 'NONE',  ( 0.000000000000000000, 0.000000000000000000, -1.000000000000000000 ) ) ;
#9555=CARTESIAN_POINT ( 'NONE',  ( -90.72413394419160682, -10.00000000000001599, 4.947285117213267469 ) ) ;
#9559=CARTESIAN_POINT ( 'NONE',  ( -90.00000000009001155, -88.00000000000000000, -1.301042606982603940E-15 ) ) ;
#9570=ORIENTED_EDGE ( 'NONE', *, *, #1792, .T. ) ;
#9572=VERTEX_POINT ( 'NONE', #3270 ) ;
#9584=ORIENTED_EDGE ( 'NONE', *, *, #2841, .F. ) ;
#9621=EDGE_LOOP ( 'NONE', ( #9155, #4029 ) ) ;
#9627=EDGE_CURVE ( 'NONE', #1507, #6567, #16136, .T. ) ;
#9652=CARTESIAN_POINT ( 'NONE',  ( -56.50000000009000445, -38.00000000000000000, 2.650000000000374278 ) ) ;
#9657=VERTEX_POINT ( 'NONE', #598 ) ;
#9662=DIRECTION ( 'NONE',  ( 0.000000000000000000, -1.000000000000000000, 0.000000000000000000 ) ) ;
#9695=CARTESIAN_POINT ( 'NONE',  ( -90.00000000009001155, -38.00000000000000000, -1.301042606982603940E-15 ) ) ;
#9696=VERTEX_POINT ( 'NONE', #5061 ) ;
#9700=ORIENTED_EDGE ( 'NONE', *, *, #342, .F. ) ;
#9723=DIRECTION ( 'NONE',  ( -0.000000000000000000, 1.000000000000000000, 0.000000000000000000 ) ) ;
#9726=CARTESIAN_POINT ( 'NONE',  ( -90.00000000009001155, -49.14213562373095812, -1.301042606982603940E-15 ) ) ;
#9729=AXIS2_PLACEMENT_3D ( 'NONE', #1527, #14856, #3144 ) ;
#9750=DIRECTION ( 'NONE',  ( 0.000000000000000000, -1.000000000000000000, 0.000000000000000000 ) ) ;
#9769=CARTESIAN_POINT ( 'NONE',  ( -79.64793068852898728, -34.99999999999999289, -31.86039329588756530 ) ) ;
#9771=VERTEX_POINT ( 'NONE', #4034 ) ;
#9775=CARTESIAN_POINT ( 'NONE',  ( -90.72413394419160682, 2.081668171172168513E-14, 4.947285117213266581 ) ) ;
#9802=EDGE_CURVE ( 'NONE', #9572, #2709, #14109, .T. ) ;
#9803=VERTEX_POINT ( 'NONE', #12588 ) ;
#9808=DIRECTION ( 'NONE',  ( -0.000000000000000000, 1.000000000000000000, -0.000000000000000000 ) ) ;
#9829=ORIENTED_EDGE ( 'NONE', *, *, #4688, .T. ) ;
#9865=FACE_BOUND ( 'NONE', #9874, .T. ) ;
#9874=EDGE_LOOP ( 'NONE', ( #16021, #6837 ) ) ;
#9879=ORIENTED_EDGE ( 'NONE', *, *, #9802, .F. ) ;
#9891=LINE ( 'NONE', #17144, #11612 ) ;
#9894=ORIENTED_EDGE ( 'NONE', *, *, #4993, .T. ) ;
#9913=AXIS2_PLACEMENT_3D ( 'NONE', #15074, #4600, #6308 ) ;
#9934=DIRECTION ( 'NONE',  ( 1.000000000000000000, 0.000000000000000000, 0.000000000000000000 ) ) ;
#9939=CARTESIAN_POINT ( 'NONE',  ( -90.38553543446691663, 1.821459649775647449E-14, -4.784491867360616268 ) ) ;
#9946=DIRECTION ( 'NONE',  ( -1.000000000000000000, 2.031314180040284764E-16, 0.000000000000000000 ) ) ;
#9954=PLANE ( 'NONE',  #6032 ) ;
#9957=CARTESIAN_POINT ( 'NONE',  ( -97.50000000009001155, -10.00000000000001599, -1.496198998029995330E-15 ) ) ;
#9985=DIRECTION ( 'NONE',  ( 0.000000000000000000, -1.000000000000000000, 0.000000000000000000 ) ) ;
#9991=CIRCLE ( 'NONE', #16388, 27.50000000000000000 ) ;
#10011=ORIENTED_EDGE ( 'NONE', *, *, #1793, .T. ) ;
#10028=CARTESIAN_POINT ( 'NONE',  ( -90.40159941089927997, 1.000000000000014655, -4.983845695167307355 ) ) ;
#10035=VERTEX_POINT ( 'NONE', #6736 ) ;
#10048=FACE_BOUND ( 'NONE', #16113, .T. ) ;
#10057=FACE_BOUND ( 'NONE', #12011, .T. ) ;
#10069=ADVANCED_FACE ( 'NONE', ( #14069 ), #1816, .F. ) ;
#10071=FACE_BOUND ( 'NONE', #15340, .T. ) ;
#10078=ORIENTED_EDGE ( 'NONE', *, *, #4993, .F. ) ;
#10116=APPLICATION_CONTEXT ( 'automotive_design' ) ;
#10118=DIRECTION ( 'NONE',  ( -0.000000000000000000, 1.000000000000000000, -0.000000000000000000 ) ) ;
#10124=EDGE_CURVE ( 'NONE', #2703, #4666, #18586, .T. ) ;
#10129=ADVANCED_FACE ( 'NONE', ( #7019 ), #12834, .F. ) ;
#10143=LINE ( 'NONE', #5580, #5161 ) ;
#10158=FACE_BOUND ( 'NONE', #12887, .T. ) ;
#10159=ORIENTED_EDGE ( 'NONE', *, *, #17962, .F. ) ;
#10195=ORIENTED_EDGE ( 'NONE', *, *, #9136, .T. ) ;
#10201=ORIENTED_EDGE ( 'NONE', *, *, #496, .T. ) ;
#10214=CIRCLE ( 'NONE', #1991, 2.649999999999992806 ) ;
#10221=PLANE ( 'NONE',  #8993 ) ;
#10278=ORIENTED_EDGE ( 'NONE', *, *, #12828, .T. ) ;
#10316=AXIS2_PLACEMENT_3D ( 'NONE', #16210, #8954, #1724 ) ;
#10336=ORIENTED_EDGE ( 'NONE', *, *, #1793, .F. ) ;
#10352=CARTESIAN_POINT ( 'NONE',  ( -117.1020693116508085, -30.00000000000000000, 19.69080595179778115 ) ) ;
#10369=ORIENTED_EDGE ( 'NONE', *, *, #4093, .F. ) ;
#10407=DIRECTION ( 'NONE',  ( -0.000000000000000000, 1.000000000000000000, -0.000000000000000000 ) ) ;
#10418=DIRECTION ( 'NONE',  ( 0.9938152567191714803, 0.000000000000000000, -0.1110460963393456596 ) ) ;
#10437=CARTESIAN_POINT ( 'NONE',  ( -117.1020693116506379, -38.00000000000000000, -19.69080595179801207 ) ) ;
#10440=ADVANCED_FACE ( 'NONE', ( #3862 ), #2233, .T. ) ;
#10470=DIRECTION ( 'NONE',  ( 0.000000000000000000, -1.000000000000000000, 0.000000000000000000 ) ) ;
#10477=VERTEX_POINT ( 'NONE', #18142 ) ;
#10491=DIRECTION ( 'NONE',  ( 0.000000000000000000, 0.000000000000000000, 1.000000000000000000 ) ) ;
#10524=AXIS2_PLACEMENT_3D ( 'NONE', #16968, #7050, #3924 ) ;
#10538=CYLINDRICAL_SURFACE ( 'NONE', #2600, 2.649999999999992806 ) ;
#10544=CARTESIAN_POINT ( 'NONE',  ( -90.00000000009003998, 1.000000000000018208, -5.746271514173173500E-15 ) ) ;
#10568=VECTOR ( 'NONE', #1453, 1000.000000000000000 ) ;
#10570=ORIENTED_EDGE ( 'NONE', *, *, #1909, .T. ) ;
#10571=CARTESIAN_POINT ( 'NONE',  ( -90.00000000009003998, 1.821459649775647449E-14, -5.746271514173173500E-15 ) ) ;
#10617=AXIS2_PLACEMENT_3D ( 'NONE', #16683, #5240, #2393 ) ;
#10642=DIRECTION ( 'NONE',  ( 0.000000000000000000, 0.000000000000000000, 1.000000000000000000 ) ) ;
#10644=ORIENTED_EDGE ( 'NONE', *, *, #12490, .T. ) ;
#10654=DIRECTION ( 'NONE',  ( -1.000000000000000000, 2.312964634635740492E-16, 0.000000000000000000 ) ) ;
#10661=CARTESIAN_POINT ( 'NONE',  ( -90.40159941089927997, -49.14213562373095812, -4.983845695167307355 ) ) ;
#10696=CARTESIAN_POINT ( 'NONE',  ( -79.64793068852927149, -34.99999999999999289, 31.86039329588764701 ) ) ;
#10698=ORIENTED_EDGE ( 'NONE', *, *, #1909, .F. ) ;
#10709=ORIENTED_EDGE ( 'NONE', *, *, #12272, .T. ) ;
#10713=FACE_OUTER_BOUND ( 'NONE', #12494, .T. ) ;
#10722=VECTOR ( 'NONE', #14031, 1000.000000000000000 ) ;
#10761=( NAMED_UNIT ( * ) SI_UNIT ( $, .STERADIAN. ) SOLID_ANGLE_UNIT ( ) );
#10813=AXIS2_PLACEMENT_3D ( 'NONE', #17392, #1387, #7096 ) ;
#10833=DIRECTION ( 'NONE',  ( -0.1586811557617541224, 0.000000000000000000, -0.9873298794253690946 ) ) ;
#10853=EDGE_CURVE ( 'NONE', #3186, #11686, #7913, .T. ) ;
#10856=EDGE_CURVE ( 'NONE', #6420, #10958, #696, .T. ) ;
#10887=VERTEX_POINT ( 'NONE', #13935 ) ;
#10893=MECHANICAL_DESIGN_GEOMETRIC_PRESENTATION_REPRESENTATION('',(#5445),#11817);
#10927=EDGE_CURVE ( 'NONE', #5529, #4919, #8412, .T. ) ;
#10939=DIRECTION ( 'NONE',  ( 0.9873298794253685395, -1.799126239882930573E-16, -0.1586811557617575918 ) ) ;
#10958=VERTEX_POINT ( 'NONE', #14985 ) ;
#10966=DIRECTION ( 'NONE',  ( 1.000000000000000000, -2.312964634635740492E-16, 0.000000000000000000 ) ) ;
#10969=DIRECTION ( 'NONE',  ( 1.000000000000000000, -2.312964634635740492E-16, 0.000000000000000000 ) ) ;
#10992=DIRECTION ( 'NONE',  ( 0.000000000000000000, -1.000000000000000000, 0.000000000000000000 ) ) ;
#11072=EDGE_CURVE ( 'NONE', #14211, #3221, #11129, .T. ) ;
#11078=FACE_OUTER_BOUND ( 'NONE', #15297, .T. ) ;
#11129=CIRCLE ( 'NONE', #18136, 7.500000000000007105 ) ;
#11140=LINE ( 'NONE', #11246, #1703 ) ;
#11163=VECTOR ( 'NONE', #16835, 1000.000000000000000 ) ;
#11169=EDGE_CURVE ( 'NONE', #4173, #18122, #14789, .T. ) ;
#11213=DIRECTION ( 'NONE',  ( 0.9938152567191714803, 0.000000000000000000, -0.1110460963393456596 ) ) ;
#11218=DIRECTION ( 'NONE',  ( -0.000000000000000000, 1.000000000000000000, 0.000000000000000000 ) ) ;
#11246=CARTESIAN_POINT ( 'NONE',  ( -90.72413394419160682, -14.11572627500821042, 4.947285117213269245 ) ) ;
#11252=AXIS2_PLACEMENT_3D ( 'NONE', #9726, #18485, #18584 ) ;
#11269=ORIENTED_EDGE ( 'NONE', *, *, #2408, .F. ) ;
#11276=LINE ( 'NONE', #17097, #17818 ) ;
#11287=EDGE_LOOP ( 'NONE', ( #671, #3042, #10369, #8807 ) ) ;
#11292=ORIENTED_EDGE ( 'NONE', *, *, #6689, .F. ) ;
#11301=DIRECTION ( 'NONE',  ( -0.08031988216184954288, 0.000000000000000000, -0.9967691390334607604 ) ) ;
#11309=ORIENTED_EDGE ( 'NONE', *, *, #12199, .T. ) ;
#11317=( LENGTH_UNIT ( ) NAMED_UNIT ( * ) SI_UNIT ( .MILLI., .METRE. ) );
#11325=ORIENTED_EDGE ( 'NONE', *, *, #11349, .F. ) ;
#11338=DIRECTION ( 'NONE',  ( 2.031314180040284764E-16, 1.000000000000000000, 1.301042606982601623E-16 ) ) ;
#11348=AXIS2_PLACEMENT_3D ( 'NONE', #9769, #1015, #16915 ) ;
#11349=EDGE_CURVE ( 'NONE', #12355, #13797, #506, .T. ) ;
#11407=SURFACE_STYLE_FILL_AREA ( #12850 ) ;
#11473=AXIS2_PLACEMENT_3D ( 'NONE', #16077, #9985, #11607 ) ;
#11492=AXIS2_PLACEMENT_3D ( 'NONE', #9695, #17134, #2360 ) ;
#11509=ORIENTED_EDGE ( 'NONE', *, *, #7771, .F. ) ;
#11515=DIRECTION ( 'NONE',  ( -0.000000000000000000, 1.000000000000000000, -0.000000000000000000 ) ) ;
#11539=CARTESIAN_POINT ( 'NONE',  ( -90.00000000009001155, 2.081668171172168513E-14, -1.301042606982603940E-15 ) ) ;
#11607=DIRECTION ( 'NONE',  ( 0.000000000000000000, 0.000000000000000000, -1.000000000000000000 ) ) ;
#11612=VECTOR ( 'NONE', #8085, 1000.000000000000000 ) ;
#11618=DIRECTION ( 'NONE',  ( -0.000000000000000000, 1.000000000000000000, -0.000000000000000000 ) ) ;
#11625=FACE_OUTER_BOUND ( 'NONE', #17241, .T. ) ;
#11631=ADVANCED_FACE ( 'NONE', ( #98 ), #14564, .T. ) ;
#11638=CARTESIAN_POINT ( 'NONE',  ( -90.00000000009001155, -88.00000000000000000, -1.301042606982603940E-15 ) ) ;
#11640=CARTESIAN_POINT ( 'NONE',  ( -117.1020693116506379, -30.00000000000000000, -22.34080595179800355 ) ) ;
#11651=CIRCLE ( 'NONE', #16511, 2.649999999999992806 ) ;
#11686=VERTEX_POINT ( 'NONE', #4469 ) ;
#11690=CARTESIAN_POINT ( 'NONE',  ( -90.00000000009001155, -13.00000000000001776, -1.691355389077386325E-15 ) ) ;
#11691=CARTESIAN_POINT ( 'NONE',  ( -90.00000000009001155, -38.00000000000000000, -40.00000000000000000 ) ) ;
#11692=VERTEX_POINT ( 'NONE', #6548 ) ;
#11698=ADVANCED_FACE ( 'NONE', ( #7979 ), #3614, .T. ) ;
#11701=( GEOMETRIC_REPRESENTATION_CONTEXT ( 3 ) GLOBAL_UNCERTAINTY_ASSIGNED_CONTEXT ( ( #5381 ) ) GLOBAL_UNIT_ASSIGNED_CONTEXT ( ( #13730, #18466, #10761 ) ) REPRESENTATION_CONTEXT ( 'NONE', 'WORKASPACE' ) );
#11719=VECTOR ( 'NONE', #15125, 1000.000000000000000 ) ;
#11731=FACE_OUTER_BOUND ( 'NONE', #17396, .T. ) ;
#11752=AXIS2_PLACEMENT_3D ( 'NONE', #601, #6698, #10966 ) ;
#11778=ORIENTED_EDGE ( 'NONE', *, *, #18088, .T. ) ;
#11783=DIRECTION ( 'NONE',  ( 1.000000000000000000, -3.469446951953611231E-16, 0.000000000000000000 ) ) ;
#11817=( GEOMETRIC_REPRESENTATION_CONTEXT ( 3 ) GLOBAL_UNCERTAINTY_ASSIGNED_CONTEXT ( ( #12240 ) ) GLOBAL_UNIT_ASSIGNED_CONTEXT ( ( #2210, #13824, #18216 ) ) REPRESENTATION_CONTEXT ( 'NONE', 'WORKASPACE' ) );
#11827=EDGE_CURVE ( 'NONE', #13797, #2843, #16466, .T. ) ;
#11830=CYLINDRICAL_SURFACE ( 'NONE', #17996, 5.000000000000004441 ) ;
#11834=ORIENTED_EDGE ( 'NONE', *, *, #11349, .T. ) ;
#11839=ORIENTED_EDGE ( 'NONE', *, *, #1219, .T. ) ;
#11840=CARTESIAN_POINT ( 'NONE',  ( -82.50000000008999734, -10.00000000000001954, -5.777138986694819161E-16 ) ) ;
#11860=EDGE_CURVE ( 'NONE', #8916, #3012, #16645, .T. ) ;
#11896=EDGE_CURVE ( 'NONE', #9267, #1277, #7206, .T. ) ;
#11900=EDGE_CURVE ( 'NONE', #15277, #8733, #17856, .T. ) ;
#11903=CARTESIAN_POINT ( 'NONE',  ( -79.64793068852927149, -34.99999999999999289, 34.51039329588763849 ) ) ;
#11926=CIRCLE ( 'NONE', #15274, 4.799999999999998934 ) ;
#11935=CARTESIAN_POINT ( 'NONE',  ( -90.70833251482494575, 1.000000000000014655, -4.949572208642815774 ) ) ;
#11938=CIRCLE ( 'NONE', #15590, 2.649999999999992806 ) ;
#11959=DIRECTION ( 'NONE',  ( 2.031314180040284764E-16, 1.000000000000000000, 1.301042606982601623E-16 ) ) ;
#11979=DIRECTION ( 'NONE',  ( 2.031314180040284764E-16, 1.000000000000000000, 1.301042606982601377E-16 ) ) ;
#11995=DIRECTION ( 'NONE',  ( -0.000000000000000000, 1.000000000000000000, -0.000000000000000000 ) ) ;
#12011=EDGE_LOOP ( 'NONE', ( #11309, #4162 ) ) ;
#12049=VERTEX_POINT ( 'NONE', #11935 ) ;
#12069=AXIS2_PLACEMENT_3D ( 'NONE', #1339, #7129, #5896 ) ;
#12108=ORIENTED_EDGE ( 'NONE', *, *, #3902, .F. ) ;
#12124=CARTESIAN_POINT ( 'NONE',  ( -117.1020693116506379, -34.99999999999999289, -19.69080595179801207 ) ) ;
#12160=EDGE_LOOP ( 'NONE', ( #9879, #8743, #16496, #738 ) ) ;
#12170=VECTOR ( 'NONE', #5197, 999.9999999999998863 ) ;
#12173=VERTEX_POINT ( 'NONE', #797 ) ;
#12182=DIRECTION ( 'NONE',  ( 0.000000000000000000, -1.000000000000000000, 0.000000000000000000 ) ) ;
#12191=VERTEX_POINT ( 'NONE', #3565 ) ;
#12199=EDGE_CURVE ( 'NONE', #6003, #11692, #9284, .T. ) ;
#12223=DIRECTION ( 'NONE',  ( 0.000000000000000000, 0.000000000000000000, -1.000000000000000000 ) ) ;
#12233=ORIENTED_EDGE ( 'NONE', *, *, #14121, .F. ) ;
#12239=VERTEX_POINT ( 'NONE', #4972 ) ;
#12240=UNCERTAINTY_MEASURE_WITH_UNIT (LENGTH_MEASURE( 1.000000000000000082E-05 ), #2210, 'distance_accuracy_value', 'NONE');
#12272=EDGE_CURVE ( 'NONE', #3012, #8916, #6859, .T. ) ;
#12287=ORIENTED_EDGE ( 'NONE', *, *, #764, .T. ) ;
#12290=SURFACE_SIDE_STYLE ('',( #11407 ) ) ;
#12355=VERTEX_POINT ( 'NONE', #10028 ) ;
#12356=DIRECTION ( 'NONE',  ( 0.9938152567191714803, 0.000000000000000000, -0.1110460963393456596 ) ) ;
#12366=FACE_OUTER_BOUND ( 'NONE', #11287, .T. ) ;
#12415=AXIS2_PLACEMENT_3D ( 'NONE', #5192, #10992, #3769 ) ;
#12437=AXIS2_PLACEMENT_3D ( 'NONE', #6374, #459, #4653 ) ;
#12442=LINE ( 'NONE', #18249, #12170 ) ;
#12453=DIRECTION ( 'NONE',  ( 0.000000000000000000, -1.000000000000000000, 0.000000000000000000 ) ) ;
#12454=ORIENTED_EDGE ( 'NONE', *, *, #13315, .F. ) ;
#12461=ORIENTED_EDGE ( 'NONE', *, *, #4455, .F. ) ;
#12490=EDGE_CURVE ( 'NONE', #9696, #2243, #8781, .T. ) ;
#12494=EDGE_LOOP ( 'NONE', ( #547, #6655, #7028, #16121 ) ) ;
#12524=DIRECTION ( 'NONE',  ( -0.000000000000000000, 1.000000000000000000, -0.000000000000000000 ) ) ;
#12546=ORIENTED_EDGE ( 'NONE', *, *, #15279, .T. ) ;
#12559=ORIENTED_EDGE ( 'NONE', *, *, #11860, .T. ) ;
#12560=CARTESIAN_POINT ( 'NONE',  ( -56.50000000009000445, -30.00000000000000000, 3.817814120399276590E-13 ) ) ;
#12588=CARTESIAN_POINT ( 'NONE',  ( -117.1020693116508085, -34.99999999999999289, 17.04080595179778967 ) ) ;
#12609=ADVANCED_BREP_SHAPE_REPRESENTATION ( '', ( #15813, #8017 ), #16855 ) ;
#12612=DIRECTION ( 'NONE',  ( 0.000000000000000000, -1.000000000000000000, 0.000000000000000000 ) ) ;
#12631=DIRECTION ( 'NONE',  ( 0.000000000000000000, -1.000000000000000000, 0.000000000000000000 ) ) ;
#12642=CARTESIAN_POINT ( 'NONE',  ( -87.76214430591549842, -10.00000000000001954, 4.471241649927994999 ) ) ;
#12647=ORIENTED_EDGE ( 'NONE', *, *, #2447, .F. ) ;
#12665=VECTOR ( 'NONE', #18778, 1000.000000000000114 ) ;
#12669=DIRECTION ( 'NONE',  ( -0.000000000000000000, 1.000000000000000000, -0.000000000000000000 ) ) ;
#12678=FACE_BOUND ( 'NONE', #16557, .T. ) ;
#12715=CYLINDRICAL_SURFACE ( 'NONE', #14307, 2.649999999999992806 ) ;
#12730=FACE_BOUND ( 'NONE', #13594, .T. ) ;
#12733=ORIENTED_EDGE ( 'NONE', *, *, #11900, .T. ) ;
#12742=ORIENTED_EDGE ( 'NONE', *, *, #3172, .F. ) ;
#12746=CARTESIAN_POINT ( 'NONE',  ( -79.64793068852898728, -38.00000000000000000, -31.86039329588756530 ) ) ;
#12752=EDGE_CURVE ( 'NONE', #14440, #5933, #4866, .T. ) ;
#12801=CARTESIAN_POINT ( 'NONE',  ( 0.000000000000000000, 0.000000000000000000, 0.000000000000000000 ) ) ;
#12825=FACE_BOUND ( 'NONE', #9621, .T. ) ;
#12828=EDGE_CURVE ( 'NONE', #7635, #9528, #17824, .T. ) ;
#12834=PLANE ( 'NONE',  #13717 ) ;
#12838=PRODUCT_DEFINITION_CONTEXT ( 'detailed design', #2206, 'design' ) ;
#12848=ORIENTED_EDGE ( 'NONE', *, *, #6751, .T. ) ;
#12850=FILL_AREA_STYLE ('',( #5046 ) ) ;
#12880=EDGE_LOOP ( 'NONE', ( #12233, #1456, #5647, #913 ) ) ;
#12887=EDGE_LOOP ( 'NONE', ( #7235, #16751 ) ) ;
#12891=CARTESIAN_POINT ( 'NONE',  ( -90.70833251482494575, -49.14213562373095812, -4.949572208642814886 ) ) ;
#12894=ORIENTED_EDGE ( 'NONE', *, *, #18667, .T. ) ;
#12907=EDGE_CURVE ( 'NONE', #13973, #9150, #11140, .T. ) ;
#12911=DIRECTION ( 'NONE',  ( 0.000000000000000000, -1.000000000000000000, 0.000000000000000000 ) ) ;
#12937=FACE_OUTER_BOUND ( 'NONE', #5731, .T. ) ;
#12965=FACE_OUTER_BOUND ( 'NONE', #17727, .T. ) ;
#12978=EDGE_CURVE ( 'NONE', #9150, #6825, #17237, .T. ) ;
#12982=CARTESIAN_POINT ( 'NONE',  ( -79.64793068852898728, -38.00000000000000000, -31.86039329588756530 ) ) ;
#12996=ORIENTED_EDGE ( 'NONE', *, *, #7018, .T. ) ;
#13025=ORIENTED_EDGE ( 'NONE', *, *, #764, .F. ) ;
#13038=ORIENTED_EDGE ( 'NONE', *, *, #4333, .T. ) ;
#13039=CARTESIAN_POINT ( 'NONE',  ( -90.00000000009001155, -38.00000000000000000, -27.50000000000000000 ) ) ;
#13046=AXIS2_PLACEMENT_3D ( 'NONE', #14795, #1747, #4794 ) ;
#13050=CARTESIAN_POINT ( 'NONE',  ( -90.00000000009001155, -38.00000000000000000, -1.301042606982603940E-15 ) ) ;
#13064=VERTEX_POINT ( 'NONE', #1428 ) ;
#13095=CARTESIAN_POINT ( 'NONE',  ( -90.00000000009001155, 1.828182762038084424E-14, -1.561251128379122243E-15 ) ) ;
#13102=DIRECTION ( 'NONE',  ( -2.031314180040284764E-16, -1.000000000000000000, -1.301042606982601377E-16 ) ) ;
#13136=VECTOR ( 'NONE', #10939, 1000.000000000000227 ) ;
#13139=CARTESIAN_POINT ( 'NONE',  ( -82.50000000008999734, -13.00000000000001954, -5.777138986694822120E-16 ) ) ;
#13149=DIRECTION ( 'NONE',  ( 0.000000000000000000, 0.000000000000000000, 1.000000000000000000 ) ) ;
#13175=ORIENTED_EDGE ( 'NONE', *, *, #42, .F. ) ;
#13195=DIRECTION ( 'NONE',  ( 0.000000000000000000, -1.000000000000000000, 0.000000000000000000 ) ) ;
#13232=DIRECTION ( 'NONE',  ( 0.000000000000000000, -1.000000000000000000, 0.000000000000000000 ) ) ;
#13241=AXIS2_PLACEMENT_3D ( 'NONE', #5468, #1079, #6985 ) ;
#13314=FACE_OUTER_BOUND ( 'NONE', #16534, .T. ) ;
#13315=EDGE_CURVE ( 'NONE', #10477, #17054, #4732, .T. ) ;
#13340=ADVANCED_FACE ( 'NONE', ( #3410 ), #6363, .T. ) ;
#13359=CARTESIAN_POINT ( 'NONE',  ( -79.64793068852927149, -30.00000000000000000, 29.21039329588765554 ) ) ;
#13365=CIRCLE ( 'NONE', #10617, 5.000000000000004441 ) ;
#13373=CARTESIAN_POINT ( 'NONE',  ( -79.64793068852898728, -30.00000000000000000, -34.51039329588756033 ) ) ;
#13392=EDGE_LOOP ( 'NONE', ( #11834, #535, #12848, #594, #14922, #12287, #15582, #15016 ) ) ;
#13407=DIRECTION ( 'NONE',  ( -0.000000000000000000, 1.000000000000000000, -0.000000000000000000 ) ) ;
#13435=ADVANCED_FACE ( 'NONE', ( #1878 ), #7679, .T. ) ;
#13442=ORIENTED_EDGE ( 'NONE', *, *, #7749, .F. ) ;
#13447=VECTOR ( 'NONE', #18367, 1000.000000000000000 ) ;
#13450=DIRECTION ( 'NONE',  ( -0.000000000000000000, 1.000000000000000000, -0.000000000000000000 ) ) ;
#13501=DIRECTION ( 'NONE',  ( 0.000000000000000000, 0.000000000000000000, -1.000000000000000000 ) ) ;
#13505=CARTESIAN_POINT ( 'NONE',  ( -90.00000000009001155, -88.00000000000000000, -1.301042606982603940E-15 ) ) ;
#13538=CARTESIAN_POINT ( 'NONE',  ( -79.64793068852898728, -34.99999999999999289, -34.51039329588756033 ) ) ;
#13551=ORIENTED_EDGE ( 'NONE', *, *, #14822, .F. ) ;
#13559=PLANE ( 'NONE',  #5866 ) ;
#13579=CARTESIAN_POINT ( 'NONE',  ( -90.00000000009001155, 1.000000000000014655, -5.000000000000005329 ) ) ;
#13594=EDGE_LOOP ( 'NONE', ( #6392, #11292 ) ) ;
#13598=ORIENTED_EDGE ( 'NONE', *, *, #1656, .T. ) ;
#13621=EDGE_LOOP ( 'NONE', ( #1364, #14058 ) ) ;
#13626=AXIS2_PLACEMENT_3D ( 'NONE', #2431, #9662, #8245 ) ;
#13627=VECTOR ( 'NONE', #7258, 1000.000000000000000 ) ;
#13661=ORIENTED_EDGE ( 'NONE', *, *, #18062, .T. ) ;
#13717=AXIS2_PLACEMENT_3D ( 'NONE', #1222, #5687, #11301 ) ;
#13723=CARTESIAN_POINT ( 'NONE',  ( -117.1020693116508085, -30.00000000000000000, 17.04080595179778967 ) ) ;
#13728=ORIENTED_EDGE ( 'NONE', *, *, #405, .F. ) ;
#13730=( LENGTH_UNIT ( ) NAMED_UNIT ( * ) SI_UNIT ( .MILLI., .METRE. ) );
#13738=ORIENTED_EDGE ( 'NONE', *, *, #17158, .T. ) ;
#13789=VERTEX_POINT ( 'NONE', #14716 ) ;
#13797=VERTEX_POINT ( 'NONE', #13579 ) ;
#13800=DIRECTION ( 'NONE',  ( -0.000000000000000000, 1.000000000000000000, -0.000000000000000000 ) ) ;
#13806=CARTESIAN_POINT ( 'NONE',  ( -90.67999921423555065, 1.821459649775647449E-14, -4.751589320297106234 ) ) ;
#13824=( NAMED_UNIT ( * ) PLANE_ANGLE_UNIT ( ) SI_UNIT ( $, .RADIAN. ) );
#13827=EDGE_CURVE ( 'NONE', #12049, #3333, #17953, .T. ) ;
#13842=DIRECTION ( 'NONE',  ( -0.000000000000000000, 1.000000000000000000, 0.000000000000000000 ) ) ;
#13851=VECTOR ( 'NONE', #1666, 1000.000000000000227 ) ;
#13865=VECTOR ( 'NONE', #7589, 1000.000000000000000 ) ;
#13869=CIRCLE ( 'NONE', #16307, 2.649999999999992806 ) ;
#13874=DIRECTION ( 'NONE',  ( 0.9938152567191714803, 0.000000000000000000, -0.1110460963393456596 ) ) ;
#13896=EDGE_LOOP ( 'NONE', ( #2533, #18590, #1204, #6224 ) ) ;
#13919=CARTESIAN_POINT ( 'NONE',  ( -90.72413394419160682, -14.11572627500821042, 4.947285117213267469 ) ) ;
#13924=AXIS2_PLACEMENT_3D ( 'NONE', #12982, #10118, #208 ) ;
#13935=CARTESIAN_POINT ( 'NONE',  ( -85.22968676783801811, 1.000000000000018208, -0.5330212624288650503 ) ) ;
#13939=DIRECTION ( 'NONE',  ( 0.000000000000000000, 0.000000000000000000, -1.000000000000000000 ) ) ;
#13951=ORIENTED_EDGE ( 'NONE', *, *, #17403, .F. ) ;
#13973=VERTEX_POINT ( 'NONE', #9555 ) ;
#13979=FACE_OUTER_BOUND ( 'NONE', #14308, .T. ) ;
#14000=CIRCLE ( 'NONE', #4275, 2.649999999999992806 ) ;
#14031=DIRECTION ( 'NONE',  ( -0.000000000000000000, 1.000000000000000000, -0.000000000000000000 ) ) ;
#14045=ADVANCED_FACE ( 'NONE', ( #1558 ), #10221, .T. ) ;
#14052=CARTESIAN_POINT ( 'NONE',  ( -90.00000000009001155, -13.00000000000001776, -5.000000000000005329 ) ) ;
#14058=ORIENTED_EDGE ( 'NONE', *, *, #15890, .T. ) ;
#14069=FACE_OUTER_BOUND ( 'NONE', #16800, .T. ) ;
#14109=LINE ( 'NONE', #2691, #8824 ) ;
#14121=EDGE_CURVE ( 'NONE', #14354, #12355, #17796, .T. ) ;
#14171=CARTESIAN_POINT ( 'NONE',  ( -90.40196296004810961, 1.745901168134654787E-14, 6.951864913735149365 ) ) ;
#14174=ORIENTED_EDGE ( 'NONE', *, *, #13315, .T. ) ;
#14211=VERTEX_POINT ( 'NONE', #11840 ) ;
#14216=DIRECTION ( 'NONE',  ( 0.000000000000000000, 0.000000000000000000, -1.000000000000000000 ) ) ;
#14228=DIRECTION ( 'NONE',  ( 0.000000000000000000, -1.000000000000000000, 0.000000000000000000 ) ) ;
#14230=ADVANCED_FACE ( 'NONE', ( #3086 ), #3366, .T. ) ;
#14257=ADVANCED_FACE ( 'NONE', ( #1738 ), #17558, .T. ) ;
#14290=AXIS2_PLACEMENT_3D ( 'NONE', #13919, #4956, #9333 ) ;
#14307=AXIS2_PLACEMENT_3D ( 'NONE', #1006, #17192, #1374 ) ;
#14308=EDGE_LOOP ( 'NONE', ( #13025, #9829, #7205, #13728 ) ) ;
#14316=DIRECTION ( 'NONE',  ( 1.000000000000000000, -2.312964634635740492E-16, 0.000000000000000000 ) ) ;
#14318=CARTESIAN_POINT ( 'NONE',  ( -117.1020693116508085, -30.00000000000000000, 19.69080595179778115 ) ) ;
#14324=DIRECTION ( 'NONE',  ( 0.000000000000000000, 0.000000000000000000, 1.000000000000000000 ) ) ;
#14354=VERTEX_POINT ( 'NONE', #597 ) ;
#14378=FACE_OUTER_BOUND ( 'NONE', #14429, .T. ) ;
#14402=LINE ( 'NONE', #11640, #10568 ) ;
#14416=DIRECTION ( 'NONE',  ( 2.031314180040284764E-16, 1.000000000000000000, 1.301042606982601377E-16 ) ) ;
#14421=DIRECTION ( 'NONE',  ( 0.000000000000000000, 0.000000000000000000, 1.000000000000000000 ) ) ;
#14427=ORIENTED_EDGE ( 'NONE', *, *, #9802, .T. ) ;
#14429=EDGE_LOOP ( 'NONE', ( #16050, #14493, #2755, #2925 ) ) ;
#14440=VERTEX_POINT ( 'NONE', #3649 ) ;
#14459=DIRECTION ( 'NONE',  ( 0.000000000000000000, -1.000000000000000000, 0.000000000000000000 ) ) ;
#14464=EDGE_CURVE ( 'NONE', #2709, #13973, #18683, .T. ) ;
#14477=AXIS2_PLACEMENT_3D ( 'NONE', #240, #13195, #3382 ) ;
#14482=AXIS2_PLACEMENT_3D ( 'NONE', #3311, #1677, #11783 ) ;
#14483=AXIS2_PLACEMENT_3D ( 'NONE', #11539, #13232, #17704 ) ;
#14490=DIRECTION ( 'NONE',  ( -0.000000000000000000, 1.000000000000000000, -0.000000000000000000 ) ) ;
#14493=ORIENTED_EDGE ( 'NONE', *, *, #1875, .T. ) ;
#14509=CARTESIAN_POINT ( 'NONE',  ( -90.38553543446691663, 1.000000000000018208, -4.784491867360616268 ) ) ;
#14514=DIRECTION ( 'NONE',  ( -0.000000000000000000, 1.000000000000000000, -0.000000000000000000 ) ) ;
#14544=CARTESIAN_POINT ( 'NONE',  ( -97.50000000009001155, -13.00000000000001599, -1.691355389077386325E-15 ) ) ;
#14560=DIRECTION ( 'NONE',  ( 0.000000000000000000, 0.000000000000000000, -1.000000000000000000 ) ) ;
#14563=ORIENTED_EDGE ( 'NONE', *, *, #10856, .T. ) ;
#14564=CYLINDRICAL_SURFACE ( 'NONE', #12069, 4.799999999999998934 ) ;
#14591=AXIS2_PLACEMENT_3D ( 'NONE', #14663, #4749, #13149 ) ;
#14592=DIRECTION ( 'NONE',  ( -0.000000000000000000, 1.000000000000000000, -0.000000000000000000 ) ) ;
#14626=EDGE_LOOP ( 'NONE', ( #4876, #426, #18230, #13551 ) ) ;
#14636=EDGE_LOOP ( 'NONE', ( #17411, #18731 ) ) ;
#14658=EDGE_CURVE ( 'NONE', #13064, #15277, #1624, .T. ) ;
#14663=CARTESIAN_POINT ( 'NONE',  ( -90.00000000009001155, -34.99999999999999289, -1.301042606982603940E-15 ) ) ;
#14680=VERTEX_POINT ( 'NONE', #11903 ) ;
#14685=ORIENTED_EDGE ( 'NONE', *, *, #2841, .T. ) ;
#14716=CARTESIAN_POINT ( 'NONE',  ( -90.00000000009001155, 2.081668171172168513E-14, -5.000000000000005329 ) ) ;
#14731=CYLINDRICAL_SURFACE ( 'NONE', #7172, 5.000000000000004441 ) ;
#14736=CIRCLE ( 'NONE', #17478, 40.00000000000000000 ) ;
#14766=DIRECTION ( 'NONE',  ( 0.000000000000000000, 0.000000000000000000, -1.000000000000000000 ) ) ;
#14789=CIRCLE ( 'NONE', #1121, 2.649999999999992806 ) ;
#14795=CARTESIAN_POINT ( 'NONE',  ( -90.40196296004810961, -14.11572627500821042, 6.951864913735147589 ) ) ;
#14822=EDGE_CURVE ( 'NONE', #14354, #4666, #9494, .T. ) ;
#14823=AXIS2_PLACEMENT_3D ( 'NONE', #3228, #4934, #12356 ) ;
#14831=VECTOR ( 'NONE', #9808, 1000.000000000000000 ) ;
#14832=DIRECTION ( 'NONE',  ( 0.000000000000000000, -1.000000000000000000, 0.000000000000000000 ) ) ;
#14836=DIRECTION ( 'NONE',  ( 0.000000000000000000, 0.000000000000000000, -1.000000000000000000 ) ) ;
#14853=AXIS2_PLACEMENT_3D ( 'NONE', #4416, #7283, #14421 ) ;
#14856=DIRECTION ( 'NONE',  ( 0.000000000000000000, -1.000000000000000000, 0.000000000000000000 ) ) ;
#14877=CARTESIAN_POINT ( 'NONE',  ( -79.64793068852898728, -30.00000000000000000, -29.21039329588757383 ) ) ;
#14895=ADVANCED_FACE ( 'NONE', ( #13979 ), #2449, .T. ) ;
#14901=PLANE ( 'NONE',  #13046 ) ;
#14905=DIRECTION ( 'NONE',  ( 0.1416665029469836024, 0.000000000000000000, 0.9899144417285627995 ) ) ;
#14922=ORIENTED_EDGE ( 'NONE', *, *, #5588, .T. ) ;
#14924=CYLINDRICAL_SURFACE ( 'NONE', #3021, 2.649999999999992806 ) ;
#14927=ORIENTED_EDGE ( 'NONE', *, *, #5588, .F. ) ;
#14928=FACE_OUTER_BOUND ( 'NONE', #15513, .T. ) ;
#14985=CARTESIAN_POINT ( 'NONE',  ( -87.76214430591549842, 2.081668171172168513E-14, 4.471241649927989670 ) ) ;
#15010=VECTOR ( 'NONE', #16478, 1000.000000000000000 ) ;
#15016=ORIENTED_EDGE ( 'NONE', *, *, #14121, .T. ) ;
#15021=CARTESIAN_POINT ( 'NONE',  ( -90.00000000009001155, -49.14213562373095812, -1.301042606982603940E-15 ) ) ;
#15023=VECTOR ( 'NONE', #14905, 1000.000000000000227 ) ;
#15027=EDGE_LOOP ( 'NONE', ( #5054, #14927, #9894, #1753 ) ) ;
#15072=ORIENTED_EDGE ( 'NONE', *, *, #9627, .F. ) ;
#15074=CARTESIAN_POINT ( 'NONE',  ( -90.00000000009001155, -88.00000000000000000, -1.301042606982603940E-15 ) ) ;
#15086=ORIENTED_EDGE ( 'NONE', *, *, #12907, .F. ) ;
#15088=CARTESIAN_POINT ( 'NONE',  ( -79.64793068852927149, -30.00000000000000000, 34.51039329588763849 ) ) ;
#15118=DIRECTION ( 'NONE',  ( -0.000000000000000000, 1.000000000000000000, -0.000000000000000000 ) ) ;
#15125=DIRECTION ( 'NONE',  ( -0.000000000000000000, 1.000000000000000000, -0.000000000000000000 ) ) ;
#15146=LINE ( 'NONE', #10661, #15010 ) ;
#15208=DIRECTION ( 'NONE',  ( 0.000000000000000000, -1.000000000000000000, 0.000000000000000000 ) ) ;
#15220=CARTESIAN_POINT ( 'NONE',  ( -90.00000000009001155, -49.14213562373095812, 5.000000000000003553 ) ) ;
#15227=CARTESIAN_POINT ( 'NONE',  ( -97.50000000009001155, -13.00000000000001599, -1.496198998029995922E-15 ) ) ;
#15266=ORIENTED_EDGE ( 'NONE', *, *, #12907, .T. ) ;
#15274=AXIS2_PLACEMENT_3D ( 'NONE', #18669, #9723, #18288 ) ;
#15277=VERTEX_POINT ( 'NONE', #3676 ) ;
#15279=EDGE_CURVE ( 'NONE', #8733, #15277, #2983, .T. ) ;
#15297=EDGE_LOOP ( 'NONE', ( #15627, #1174, #10201, #15835 ) ) ;
#15340=EDGE_LOOP ( 'NONE', ( #10278, #4973 ) ) ;
#15414=AXIS2_PLACEMENT_3D ( 'NONE', #9429, #16485, #3442 ) ;
#15487=CARTESIAN_POINT ( 'NONE',  ( -117.1020693116506379, -34.99999999999999289, -17.04080595179801705 ) ) ;
#15494=CARTESIAN_POINT ( 'NONE',  ( -117.1020693116508085, -34.99999999999999289, 22.34080595179777262 ) ) ;
#15513=EDGE_LOOP ( 'NONE', ( #6659, #9346, #3933, #6090 ) ) ;
#15547=EDGE_LOOP ( 'NONE', ( #5215, #3977, #12546, #4830 ) ) ;
#15554=CARTESIAN_POINT ( 'NONE',  ( -90.00000000009001155, -10.00000000000001776, -1.301042606982605912E-15 ) ) ;
#15560=CARTESIAN_POINT ( 'NONE',  ( -82.50000000008999734, -13.00000000000001954, -7.728702897168715310E-16 ) ) ;
#15582=ORIENTED_EDGE ( 'NONE', *, *, #18327, .T. ) ;
#15590=AXIS2_PLACEMENT_3D ( 'NONE', #3707, #12182, #3338 ) ;
#15627=ORIENTED_EDGE ( 'NONE', *, *, #1875, .F. ) ;
#15644=DIRECTION ( 'NONE',  ( 0.000000000000000000, -1.000000000000000000, 0.000000000000000000 ) ) ;
#15688=CARTESIAN_POINT ( 'NONE',  ( -56.50000000009000445, -38.00000000000000000, 3.817814120399276590E-13 ) ) ;
#15729=CARTESIAN_POINT ( 'NONE',  ( -90.00000000009001155, -88.00000000000000000, -27.50000000000000000 ) ) ;
#15794=DIRECTION ( 'NONE',  ( 0.000000000000000000, -1.000000000000000000, 0.000000000000000000 ) ) ;
#15804=SURFACE_STYLE_USAGE ( .BOTH. , #12290 ) ;
#15813=MANIFOLD_SOLID_BREP ( 'M5 Clearance Hole2', #3143 ) ;
#15835=ORIENTED_EDGE ( 'NONE', *, *, #3137, .F. ) ;
#15848=PRODUCT_CONTEXT ( 'NONE', #10116, 'mechanical' ) ;
#15858=CARTESIAN_POINT ( 'NONE',  ( -90.00000000009001155, -10.00000000000001776, -1.301042606982605912E-15 ) ) ;
#15879=CARTESIAN_POINT ( 'NONE',  ( -90.00000000009001155, -38.00000000000000000, -1.301042606982603940E-15 ) ) ;
#15890=EDGE_CURVE ( 'NONE', #9389, #13064, #9991, .T. ) ;
#15903=LINE ( 'NONE', #18478, #14831 ) ;
#15923=EDGE_LOOP ( 'NONE', ( #7224, #8627 ) ) ;
#15954=FACE_OUTER_BOUND ( 'NONE', #14636, .T. ) ;
#15964=FACE_BOUND ( 'NONE', #9251, .T. ) ;
#15990=CYLINDRICAL_SURFACE ( 'NONE', #841, 2.649999999999992806 ) ;
#16009=CIRCLE ( 'NONE', #7791, 5.000000000000004441 ) ;
#16021=ORIENTED_EDGE ( 'NONE', *, *, #342, .T. ) ;
#16050=ORIENTED_EDGE ( 'NONE', *, *, #10853, .F. ) ;
#16077=CARTESIAN_POINT ( 'NONE',  ( -90.00000000009001155, -88.00000000000000000, -1.301042606982603940E-15 ) ) ;
#16113=EDGE_LOOP ( 'NONE', ( #14427, #2426, #17689, #16159, #2379 ) ) ;
#16121=ORIENTED_EDGE ( 'NONE', *, *, #9442, .F. ) ;
#16136=LINE ( 'NONE', #13373, #2760 ) ;
#16142=ORIENTED_EDGE ( 'NONE', *, *, #11896, .F. ) ;
#16159=ORIENTED_EDGE ( 'NONE', *, *, #11896, .T. ) ;
#16183=DIRECTION ( 'NONE',  ( -2.031314180040284764E-16, -1.000000000000000000, -1.301042606982601377E-16 ) ) ;
#16210=CARTESIAN_POINT ( 'NONE',  ( -90.00000000009001155, -34.99999999999999289, -1.301042606982603940E-15 ) ) ;
#16287=CARTESIAN_POINT ( 'NONE',  ( -79.64793068852898728, -30.00000000000000000, -31.86039329588756530 ) ) ;
#16294=CARTESIAN_POINT ( 'NONE',  ( -90.00000000009001155, -49.14213562373095812, -1.301042606982603940E-15 ) ) ;
#16307=AXIS2_PLACEMENT_3D ( 'NONE', #17385, #12911, #2621 ) ;
#16322=ORIENTED_EDGE ( 'NONE', *, *, #395, .T. ) ;
#16347=AXIS2_PLACEMENT_3D ( 'NONE', #13050, #11618, #2951 ) ;
#16379=AXIS2_PLACEMENT_3D ( 'NONE', #9388, #15208, #2151 ) ;
#16383=CARTESIAN_POINT ( 'NONE',  ( -87.43997332177200121, -14.11572627500821042, 6.475821446449874230 ) ) ;
#16388=AXIS2_PLACEMENT_3D ( 'NONE', #11638, #4394, #14216 ) ;
#16415=CIRCLE ( 'NONE', #14591, 5.000000000000004441 ) ;
#16444=CYLINDRICAL_SURFACE ( 'NONE', #4205, 2.649999999999992806 ) ;
#16459=EDGE_CURVE ( 'NONE', #1893, #10035, #14736, .T. ) ;
#16466=LINE ( 'NONE', #3419, #17272 ) ;
#16478=DIRECTION ( 'NONE',  ( 0.000000000000000000, -1.000000000000000000, 0.000000000000000000 ) ) ;
#16485=DIRECTION ( 'NONE',  ( 0.000000000000000000, -1.000000000000000000, 0.000000000000000000 ) ) ;
#16489=DIRECTION ( 'NONE',  ( -0.000000000000000000, 1.000000000000000000, -0.000000000000000000 ) ) ;
#16496=ORIENTED_EDGE ( 'NONE', *, *, #395, .F. ) ;
#16511=AXIS2_PLACEMENT_3D ( 'NONE', #10437, #16628, #3593 ) ;
#16521=DIRECTION ( 'NONE',  ( 0.9938152567191714803, 0.000000000000000000, -0.1110460963393456596 ) ) ;
#16534=EDGE_LOOP ( 'NONE', ( #12996, #17853, #8094, #12454 ) ) ;
#16557=EDGE_LOOP ( 'NONE', ( #9584, #12742 ) ) ;
#16615=AXIS2_PLACEMENT_3D ( 'NONE', #16383, #3514, #10833 ) ;
#16616=EDGE_CURVE ( 'NONE', #12191, #1507, #7988, .T. ) ;
#16628=DIRECTION ( 'NONE',  ( -0.000000000000000000, 1.000000000000000000, -0.000000000000000000 ) ) ;
#16645=CIRCLE ( 'NONE', #846, 2.649999999999992806 ) ;
#16655=DIRECTION ( 'NONE',  ( -0.000000000000000000, 1.000000000000000000, -0.000000000000000000 ) ) ;
#16683=CARTESIAN_POINT ( 'NONE',  ( -90.00000000009001155, 1.000000000000014655, -1.301042606982603940E-15 ) ) ;
#16686=PRESENTATION_STYLE_ASSIGNMENT (( #15804 ) ) ;
#16701=CARTESIAN_POINT ( 'NONE',  ( -117.1020693116506379, -38.00000000000000000, -19.69080595179801207 ) ) ;
#16706=CIRCLE ( 'NONE', #10316, 5.000000000000004441 ) ;
#16751=ORIENTED_EDGE ( 'NONE', *, *, #8424, .T. ) ;
#16768=ADVANCED_FACE ( 'NONE', ( #3276 ), #13559, .F. ) ;
#16772=CYLINDRICAL_SURFACE ( 'NONE', #18157, 2.649999999999992806 ) ;
#16795=ORIENTED_EDGE ( 'NONE', *, *, #7218, .T. ) ;
#16800=EDGE_LOOP ( 'NONE', ( #15072, #17156, #13738, #9111 ) ) ;
#16835=DIRECTION ( 'NONE',  ( 0.000000000000000000, -1.000000000000000000, 0.000000000000000000 ) ) ;
#16836=EDGE_CURVE ( 'NONE', #9267, #13789, #990, .T. ) ;
#16837=ORIENTED_EDGE ( 'NONE', *, *, #11900, .F. ) ;
#16846=VECTOR ( 'NONE', #17094, 1000.000000000000000 ) ;
#16855=( GEOMETRIC_REPRESENTATION_CONTEXT ( 3 ) GLOBAL_UNCERTAINTY_ASSIGNED_CONTEXT ( ( #826 ) ) GLOBAL_UNIT_ASSIGNED_CONTEXT ( ( #11317, #3539, #4088 ) ) REPRESENTATION_CONTEXT ( 'NONE', 'WORKASPACE' ) );
#16880=AXIS2_PLACEMENT_3D ( 'NONE', #10544, #9205, #6073 ) ;
#16898=CARTESIAN_POINT ( 'NONE',  ( -90.00000000009003998, 1.000000000000018208, -5.746271514173173500E-15 ) ) ;
#16900=AXIS2_PLACEMENT_3D ( 'NONE', #12124, #2306, #13939 ) ;
#16915=DIRECTION ( 'NONE',  ( 0.000000000000000000, 0.000000000000000000, -1.000000000000000000 ) ) ;
#16917=ORIENTED_EDGE ( 'NONE', *, *, #12978, .T. ) ;
#16968=CARTESIAN_POINT ( 'NONE',  ( -56.50000000009000445, -38.00000000000000000, 3.817814120399276590E-13 ) ) ;
#17004=ORIENTED_EDGE ( 'NONE', *, *, #16836, .F. ) ;
#17019=CIRCLE ( 'NONE', #14482, 5.000000000000004441 ) ;
#17032=AXIS2_PLACEMENT_3D ( 'NONE', #6820, #12631, #18436 ) ;
#17051=ORIENTED_EDGE ( 'NONE', *, *, #1681, .T. ) ;
#17054=VERTEX_POINT ( 'NONE', #2696 ) ;
#17055=ADVANCED_FACE ( 'NONE', ( #11731 ), #17275, .F. ) ;
#17078=CARTESIAN_POINT ( 'NONE',  ( -90.00000000009001155, -13.00000000000001776, -1.691355389077386325E-15 ) ) ;
#17081=ORIENTED_EDGE ( 'NONE', *, *, #6751, .F. ) ;
#17088=CARTESIAN_POINT ( 'NONE',  ( -90.00000000009001155, -34.99999999999999289, -1.301042606982603940E-15 ) ) ;
#17094=DIRECTION ( 'NONE',  ( 2.031314180040284764E-16, 1.000000000000000000, 1.301042606982601377E-16 ) ) ;
#17097=CARTESIAN_POINT ( 'NONE',  ( -94.77031323234206184, 1.000000000000018208, 0.5330212624288539480 ) ) ;
#17108=FACE_OUTER_BOUND ( 'NONE', #5301, .T. ) ;
#17125=AXIS2_PLACEMENT_3D ( 'NONE', #12746, #17131, #4077 ) ;
#17130=LINE ( 'NONE', #1645, #2969 ) ;
#17131=DIRECTION ( 'NONE',  ( -0.000000000000000000, 1.000000000000000000, -0.000000000000000000 ) ) ;
#17134=DIRECTION ( 'NONE',  ( 0.000000000000000000, -1.000000000000000000, 0.000000000000000000 ) ) ;
#17144=CARTESIAN_POINT ( 'NONE',  ( -117.1020693116506379, -30.00000000000000000, -17.04080595179801705 ) ) ;
#17156=ORIENTED_EDGE ( 'NONE', *, *, #16616, .F. ) ;
#17158=EDGE_CURVE ( 'NONE', #12191, #3837, #7711, .T. ) ;
#17180=ADVANCED_FACE ( 'NONE', ( #6008 ), #11830, .T. ) ;
#17182=DIRECTION ( 'NONE',  ( -0.08031988216184954288, 0.000000000000000000, -0.9967691390334607604 ) ) ;
#17192=DIRECTION ( 'NONE',  ( -0.000000000000000000, 1.000000000000000000, -0.000000000000000000 ) ) ;
#17195=FACE_OUTER_BOUND ( 'NONE', #6199, .T. ) ;
#17218=FACE_BOUND ( 'NONE', #8355, .T. ) ;
#17237=CIRCLE ( 'NONE', #14483, 5.000000000000004441 ) ;
#17241=EDGE_LOOP ( 'NONE', ( #18777, #948 ) ) ;
#17272=VECTOR ( 'NONE', #9213, 1000.000000000000000 ) ;
#17275=CYLINDRICAL_SURFACE ( 'NONE', #1867, 2.649999999999992806 ) ;
#17296=CARTESIAN_POINT ( 'NONE',  ( -90.00000000009001155, -88.00000000000000000, -27.50000000000000000 ) ) ;
#17326=ORIENTED_EDGE ( 'NONE', *, *, #7697, .F. ) ;
#17349=ORIENTED_EDGE ( 'NONE', *, *, #16616, .T. ) ;
#17385=CARTESIAN_POINT ( 'NONE',  ( -117.1020693116506379, -34.99999999999999289, -19.69080595179801207 ) ) ;
#17392=CARTESIAN_POINT ( 'NONE',  ( -90.00000000009001155, -13.00000000000001776, -1.691355389077386325E-15 ) ) ;
#17396=EDGE_LOOP ( 'NONE', ( #7251, #17672, #12647, #17326 ) ) ;
#17403=EDGE_CURVE ( 'NONE', #17733, #2703, #11926, .T. ) ;
#17411=ORIENTED_EDGE ( 'NONE', *, *, #1792, .F. ) ;
#17471=CARTESIAN_POINT ( 'NONE',  ( -90.00000000009003998, 1.000000000000018208, -5.746271514173173500E-15 ) ) ;
#17478=AXIS2_PLACEMENT_3D ( 'NONE', #2258, #17981, #7976 ) ;
#17494=DIRECTION ( 'NONE',  ( 2.031314180040284764E-16, 1.000000000000000000, 1.301042606982601377E-16 ) ) ;
#17534=CARTESIAN_POINT ( 'NONE',  ( -90.00000000009001155, -88.00000000000000000, 27.50000000000000000 ) ) ;
#17542=VECTOR ( 'NONE', #7505, 1000.000000000000000 ) ;
#17558=CYLINDRICAL_SURFACE ( 'NONE', #7788, 5.000000000000004441 ) ;
#17613=AXIS2_PLACEMENT_3D ( 'NONE', #3038, #2932, #14836 ) ;
#17664=CARTESIAN_POINT ( 'NONE',  ( -90.00000000009003998, 1.821459649775647449E-14, -5.746271514173173500E-15 ) ) ;
#17672=ORIENTED_EDGE ( 'NONE', *, *, #996, .T. ) ;
#17685=ORIENTED_EDGE ( 'NONE', *, *, #18679, .F. ) ;
#17687=ADVANCED_FACE ( 'NONE', ( #18075 ), #564, .T. ) ;
#17689=ORIENTED_EDGE ( 'NONE', *, *, #2408, .T. ) ;
#17702=DIRECTION ( 'NONE',  ( 1.000000000000000000, -3.469446951953611231E-16, 0.000000000000000000 ) ) ;
#17704=DIRECTION ( 'NONE',  ( 0.000000000000000000, 0.000000000000000000, -1.000000000000000000 ) ) ;
#17727=EDGE_LOOP ( 'NONE', ( #9416, #13038 ) ) ;
#17733=VERTEX_POINT ( 'NONE', #9132 ) ;
#17736=EDGE_CURVE ( 'NONE', #2243, #14680, #11938, .T. ) ;
#17758=ORIENTED_EDGE ( 'NONE', *, *, #9627, .T. ) ;
#17796=LINE ( 'NONE', #14509, #3846 ) ;
#17818=VECTOR ( 'NONE', #4047, 1000.000000000000000 ) ;
#17824=CIRCLE ( 'NONE', #10524, 2.649999999999992806 ) ;
#17853=ORIENTED_EDGE ( 'NONE', *, *, #12752, .T. ) ;
#17856=CIRCLE ( 'NONE', #11492, 27.50000000000000000 ) ;
#17865=ORIENTED_EDGE ( 'NONE', *, *, #5986, .F. ) ;
#17882=DIRECTION ( 'NONE',  ( -0.000000000000000000, 1.000000000000000000, -0.000000000000000000 ) ) ;
#17887=PRODUCT ( 'motor', 'motor', '', ( #15848 ) ) ;
#17908=ORIENTED_EDGE ( 'NONE', *, *, #4052, .F. ) ;
#17917=DIRECTION ( 'NONE',  ( 0.000000000000000000, 0.000000000000000000, 1.000000000000000000 ) ) ;
#17947=ORIENTED_EDGE ( 'NONE', *, *, #18062, .F. ) ;
#17953=LINE ( 'NONE', #6052, #13851 ) ;
#17954=CARTESIAN_POINT ( 'NONE',  ( -90.00000000009001155, -10.00000000000001599, -5.000000000000005329 ) ) ;
#17961=ORIENTED_EDGE ( 'NONE', *, *, #1845, .F. ) ;
#17962=EDGE_CURVE ( 'NONE', #5480, #1893, #258, .T. ) ;
#17981=DIRECTION ( 'NONE',  ( 0.000000000000000000, -1.000000000000000000, 0.000000000000000000 ) ) ;
#17996=AXIS2_PLACEMENT_3D ( 'NONE', #16294, #3251, #17917 ) ;
#18000=LINE ( 'NONE', #13723, #8431 ) ;
#18006=FACE_OUTER_BOUND ( 'NONE', #1737, .T. ) ;
#18031=LINE ( 'NONE', #4978, #15023 ) ;
#18062=EDGE_CURVE ( 'NONE', #5529, #3221, #2923, .T. ) ;
#18075=FACE_OUTER_BOUND ( 'NONE', #8544, .T. ) ;
#18078=FACE_OUTER_BOUND ( 'NONE', #7051, .T. ) ;
#18088=EDGE_CURVE ( 'NONE', #11686, #3186, #11651, .T. ) ;
#18122=VERTEX_POINT ( 'NONE', #4829 ) ;
#18136=AXIS2_PLACEMENT_3D ( 'NONE', #2694, #1075, #14316 ) ;
#18142=CARTESIAN_POINT ( 'NONE',  ( -90.00000000009001155, -34.99999999999999289, 5.000000000000003553 ) ) ;
#18157=AXIS2_PLACEMENT_3D ( 'NONE', #5141, #9521, #8099 ) ;
#18162=DIRECTION ( 'NONE',  ( -0.000000000000000000, 1.000000000000000000, -0.000000000000000000 ) ) ;
#18183=AXIS2_PLACEMENT_3D ( 'NONE', #18800, #14228, #4232 ) ;
#18192=FACE_OUTER_BOUND ( 'NONE', #13896, .T. ) ;
#18205=EDGE_CURVE ( 'NONE', #6567, #3837, #706, .T. ) ;
#18211=CIRCLE ( 'NONE', #7252, 5.000000000000004441 ) ;
#18216=( NAMED_UNIT ( * ) SI_UNIT ( $, .STERADIAN. ) SOLID_ANGLE_UNIT ( ) );
#18217=DIRECTION ( 'NONE',  ( -0.1586811557617541502, 1.606889522083424400E-16, -0.9873298794253692057 ) ) ;
#18230=ORIENTED_EDGE ( 'NONE', *, *, #10124, .T. ) ;
#18249=CARTESIAN_POINT ( 'NONE',  ( -90.72413394419160682, 1.778525910263251795E-14, 4.947285117213269245 ) ) ;
#18288=DIRECTION ( 'NONE',  ( 0.9938152567191714803, 0.000000000000000000, -0.1110460963393456596 ) ) ;
#18305=CARTESIAN_POINT ( 'NONE',  ( -87.43997332177200121, 1.691927380938166737E-14, 6.475821446449876007 ) ) ;
#18308=DIRECTION ( 'NONE',  ( -2.031314180040284764E-16, -1.000000000000000000, -1.301042606982601377E-16 ) ) ;
#18311=ORIENTED_EDGE ( 'NONE', *, *, #1681, .F. ) ;
#18312=CARTESIAN_POINT ( 'NONE',  ( -87.43997332177200121, 1.691927380938166737E-14, 6.475821446449876007 ) ) ;
#18327=EDGE_CURVE ( 'NONE', #10887, #14354, #4372, .T. ) ;
#18336=ORIENTED_EDGE ( 'NONE', *, *, #11072, .T. ) ;
#18367=DIRECTION ( 'NONE',  ( 0.000000000000000000, -1.000000000000000000, 0.000000000000000000 ) ) ;
#18383=DIRECTION ( 'NONE',  ( -0.000000000000000000, 1.000000000000000000, -0.000000000000000000 ) ) ;
#18402=CARTESIAN_POINT ( 'NONE',  ( -117.1020693116508085, -30.00000000000000000, 22.34080595179777262 ) ) ;
#18427=CARTESIAN_POINT ( 'NONE',  ( -117.1020693116508085, -38.00000000000000000, 22.34080595179777262 ) ) ;
#18436=DIRECTION ( 'NONE',  ( 0.000000000000000000, 0.000000000000000000, -1.000000000000000000 ) ) ;
#18466=( NAMED_UNIT ( * ) PLANE_ANGLE_UNIT ( ) SI_UNIT ( $, .RADIAN. ) );
#18478=CARTESIAN_POINT ( 'NONE',  ( -90.00000000009001155, -49.14213562373095812, 5.000000000000003553 ) ) ;
#18485=DIRECTION ( 'NONE',  ( -0.000000000000000000, 1.000000000000000000, -0.000000000000000000 ) ) ;
#18496=VECTOR ( 'NONE', #14514, 1000.000000000000000 ) ;
#18525=DIRECTION ( 'NONE',  ( -0.08031988216184954288, 0.000000000000000000, -0.9967691390334607604 ) ) ;
#18546=CARTESIAN_POINT ( 'NONE',  ( -90.38553543446691663, 1.000000000000018208, -4.784491867360616268 ) ) ;
#18584=DIRECTION ( 'NONE',  ( 0.000000000000000000, 0.000000000000000000, 1.000000000000000000 ) ) ;
#18586=CIRCLE ( 'NONE', #6723, 4.799999999999998934 ) ;
#18590=ORIENTED_EDGE ( 'NONE', *, *, #8831, .F. ) ;
#18603=EDGE_CURVE ( 'NONE', #6825, #4781, #18031, .T. ) ;
#18667=EDGE_CURVE ( 'NONE', #13789, #10958, #3761, .T. ) ;
#18669=CARTESIAN_POINT ( 'NONE',  ( -90.00000000009003998, 1.821459649775647449E-14, -5.746271514173173500E-15 ) ) ;
#18679=EDGE_CURVE ( 'NONE', #4919, #14211, #6507, .T. ) ;
#18683=LINE ( 'NONE', #7151, #12665 ) ;
#18711=CARTESIAN_POINT ( 'NONE',  ( -90.00000000009001155, -13.00000000000001776, -1.301042606982603940E-15 ) ) ;
#18731=ORIENTED_EDGE ( 'NONE', *, *, #16459, .F. ) ;
#18741=DIRECTION ( 'NONE',  ( 0.000000000000000000, 0.000000000000000000, 1.000000000000000000 ) ) ;
#18777=ORIENTED_EDGE ( 'NONE', *, *, #5972, .F. ) ;
#18778=DIRECTION ( 'NONE',  ( -0.1586811557617541224, 1.606889522083433522E-16, -0.9873298794253690946 ) ) ;
#18800=CARTESIAN_POINT ( 'NONE',  ( -90.00000000009001155, 2.081668171172168513E-14, -1.301042606982603940E-15 ) ) ;
#18884=COLOUR_RGB('Off White',0.89,0.88,0.83);
#18885=FILL_AREA_STYLE_COLOUR('',#18884);
#18886=FILL_AREA_STYLE('',(#18885));
#18887=SURFACE_STYLE_FILL_AREA(#18886);
#18888=SURFACE_SIDE_STYLE('',(#18887));
#18889=SURFACE_STYLE_USAGE(.BOTH.,#18888);
#18890=PRESENTATION_STYLE_ASSIGNMENT((#18889));
ENDSEC;
END-ISO-10303-21;
